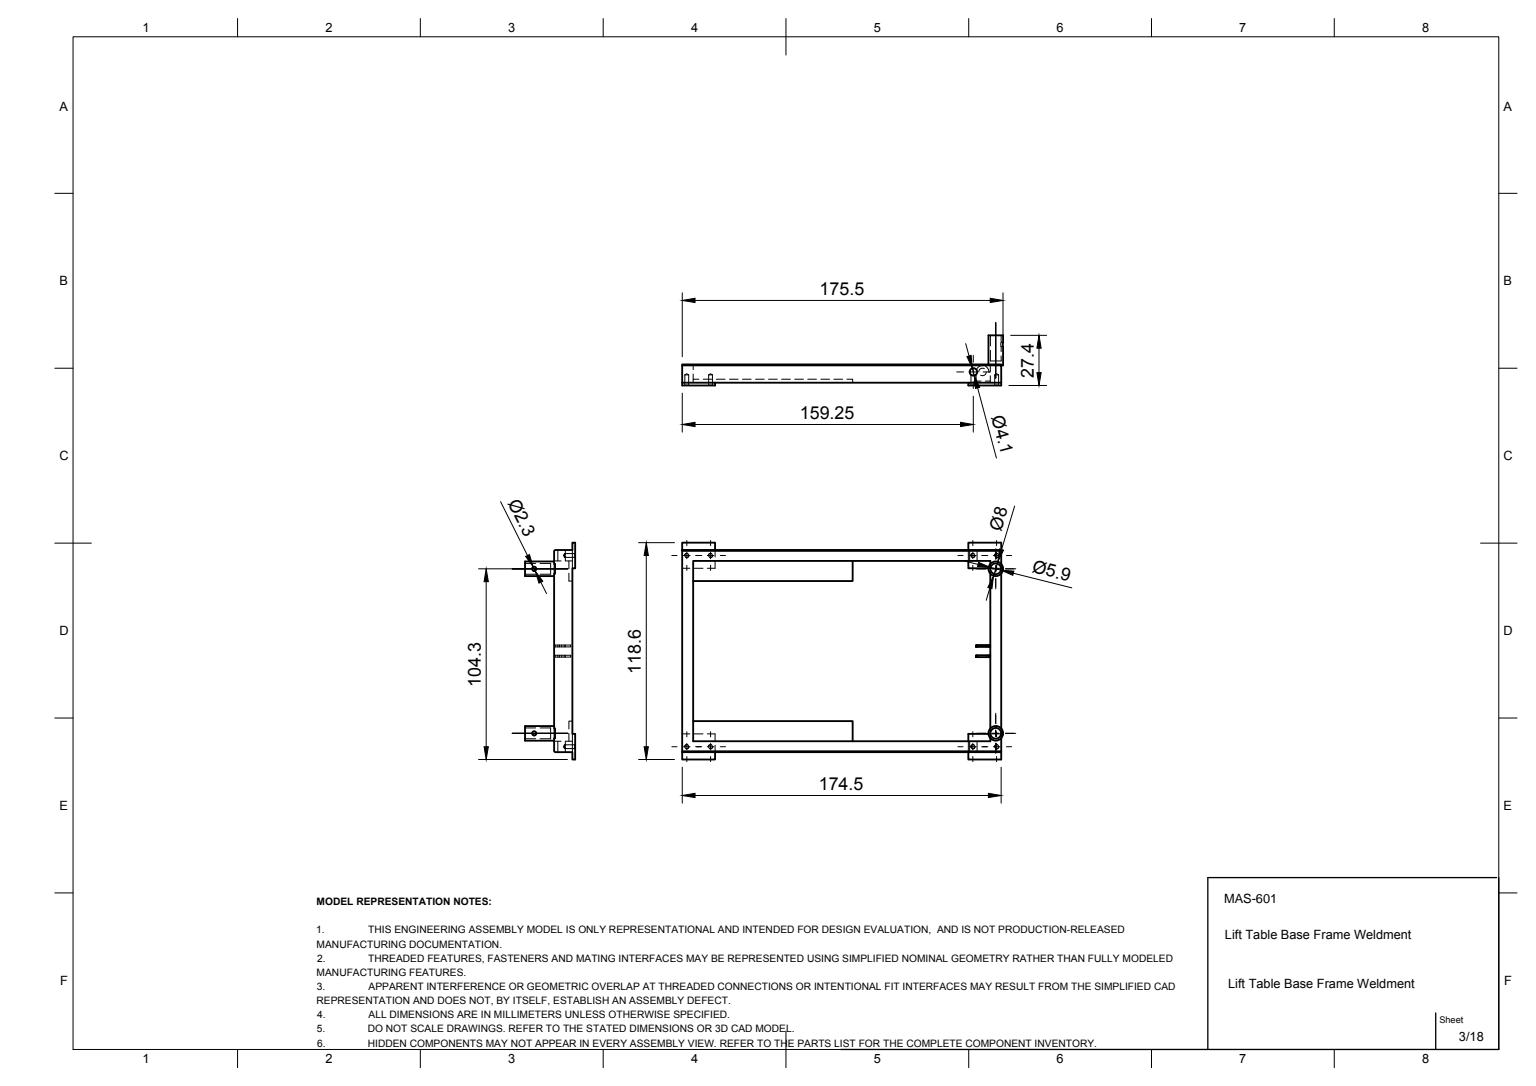
ISO-10303-21;
HEADER;
FILE_DESCRIPTION((''),'2;1');
FILE_NAME('Lift Table Base Frame Weldment.step','2026-10-06T07:37:42+05:00',(''),(''),'','','');
FILE_SCHEMA (('AUTOMOTIVE_DESIGN { 1 0 10303 214 3 1 1 }'));
ENDSEC;
DATA;
#10=MECHANICAL_DESIGN_GEOMETRIC_PRESENTATION_REPRESENTATION('',(#373),#18757);
#339=SHAPE_REPRESENTATION_RELATIONSHIP('SRR','None',#18857,#356) ;
#356=ADVANCED_BREP_SHAPE_REPRESENTATION('',(#390),#18740) ;
#373=STYLED_ITEM('',(#18951),#390) ;
#390=MANIFOLD_SOLID_BREP('Lift Table Base Frame Weldment',#9542) ;
#407=B_SPLINE_CURVE_WITH_KNOTS('',3,(#13518,#13519,#13520,#13521,#13522,
#13523,#13524,#13525,#13526,#13527,#13528,#13529,#13530,#13531,#13532,#13533,
#13534,#13535,#13536,#13537,#13538,#13539,#13540,#13541,#13542,#13543,#13544,
#13545,#13546,#13547,#13548,#13549,#13550,#13551,#13552),.UNSPECIFIED.,
 .F.,.F.,(4,2,2,2,2,2,2,2,3,2,2,2,2,2,2,2,4),(0.344577820460866,0.365980688401704,
0.406814525836436,0.448673337816236,0.490532149796036,0.530173091565364,
0.569814033334692,0.610053867634319,0.650293701933945,0.690533536233571,
0.730773370533197,0.770414312302526,0.810055254071854,0.851914066051654,
0.893772878031454,0.934606715466186,0.956009583407023),.UNSPECIFIED.) ;
#408=B_SPLINE_CURVE_WITH_KNOTS('',3,(#13564,#13565,#13566,#13567,#13568,
#13569,#13570,#13571,#13572,#13573,#13574,#13575,#13576,#13577,#13578,#13579,
#13580,#13581,#13582,#13583,#13584,#13585,#13586,#13587,#13588,#13589,#13590,
#13591,#13592,#13593,#13594,#13595,#13596,#13597,#13598),.UNSPECIFIED.,
 .F.,.F.,(4,2,2,2,2,2,2,2,3,2,2,2,2,2,2,2,4),(0.344577820460867,0.365980688401704,
0.406814525836436,0.448673337816236,0.490532149796036,0.530173091565364,
0.569814033334692,0.610053867634319,0.650293701933945,0.690533536233571,
0.730773370533197,0.770414312302526,0.810055254071854,0.851914066051654,
0.893772878031454,0.934606715466186,0.956009583407027),.UNSPECIFIED.) ;
#409=B_SPLINE_CURVE_WITH_KNOTS('',3,(#13629,#13630,#13631,#13632,#13633,
#13634,#13635),.UNSPECIFIED.,.F.,.F.,(4,3,4),(-0.0190556203788655,0.,0.0190556203788683),
 .UNSPECIFIED.) ;
#410=B_SPLINE_CURVE_WITH_KNOTS('',3,(#13646,#13647,#13648,#13649,#13650,
#13651,#13652),.UNSPECIFIED.,.F.,.F.,(4,3,4),(-0.019055620378868,0.,0.0190556203788661),
 .UNSPECIFIED.) ;
#411=B_SPLINE_CURVE_WITH_KNOTS('',3,(#13665,#13666,#13667,#13668,#13669,
#13670,#13671,#13672,#13673,#13674),.UNSPECIFIED.,.F.,.F.,(4,2,2,2,4),(0.,
0.0435910279952308,0.0871820559904617,0.130762210503654,0.174342365016846),
 .UNSPECIFIED.) ;
#412=B_SPLINE_CURVE_WITH_KNOTS('',3,(#13675,#13676,#13677,#13678,#13679,
#13680,#13681,#13682,#13683,#13684,#13685,#13686,#13687,#13688,#13689,#13690,
#13691,#13692,#13693,#13694,#13695,#13696,#13697,#13698,#13699,#13700),
 .UNSPECIFIED.,.F.,.F.,(4,2,2,2,2,2,2,2,2,2,2,2,4),(0.174342365016846,0.217922519530038,
0.261502674043231,0.305093702038462,0.348684730033692,0.392275758028923,
0.435866786024154,0.479446940537346,0.523027095050539,0.566607249563731,
0.610187404076923,0.653778432072154,0.697369460067385),.UNSPECIFIED.) ;
#413=B_SPLINE_CURVE_WITH_KNOTS('',3,(#13704,#13705,#13706,#13707,#13708,
#13709,#13710,#13711,#13712,#13713),.UNSPECIFIED.,.F.,.F.,(4,2,2,2,4),(0.,
0.0438474980267263,0.0876949960534527,0.131502815085544,0.175310634117636),
 .UNSPECIFIED.) ;
#414=B_SPLINE_CURVE_WITH_KNOTS('',3,(#13714,#13715,#13716,#13717,#13718,
#13719,#13720,#13721,#13722,#13723,#13724,#13725,#13726,#13727,#13728,#13729,
#13730,#13731,#13732,#13733,#13734,#13735,#13736,#13737,#13738,#13739),
 .UNSPECIFIED.,.F.,.F.,(4,2,2,2,2,2,2,2,2,2,2,2,4),(0.175310634117636,0.219118453149728,
0.26292627218182,0.306773770208546,0.350621268235272,0.394468766261999,
0.438316264288725,0.482124083320817,0.525931902352908,0.569739721385,0.613547540417092,
0.657395038443818,0.701242536470545),.UNSPECIFIED.) ;
#415=B_SPLINE_CURVE_WITH_KNOTS('',3,(#13750,#13751,#13752,#13753,#13754,
#13755,#13756,#13757,#13758,#13759),.UNSPECIFIED.,.F.,.F.,(4,2,2,2,4),(0.,
0.0435910279952308,0.0871820559904617,0.130762210503654,0.174342365016846),
 .UNSPECIFIED.) ;
#416=B_SPLINE_CURVE_WITH_KNOTS('',3,(#13760,#13761,#13762,#13763,#13764,
#13765,#13766,#13767,#13768,#13769,#13770,#13771,#13772,#13773,#13774,#13775,
#13776,#13777,#13778,#13779,#13780,#13781,#13782,#13783,#13784,#13785),
 .UNSPECIFIED.,.F.,.F.,(4,2,2,2,2,2,2,2,2,2,2,2,4),(0.174342365016846,0.217922519530038,
0.261502674043231,0.305093702038462,0.348684730033692,0.392275758028923,
0.435866786024154,0.479446940537346,0.523027095050539,0.566607249563731,
0.610187404076923,0.653778432072154,0.697369460067385),.UNSPECIFIED.) ;
#417=B_SPLINE_CURVE_WITH_KNOTS('',3,(#13789,#13790,#13791,#13792,#13793,
#13794,#13795,#13796,#13797,#13798),.UNSPECIFIED.,.F.,.F.,(4,2,2,2,4),(0.,
0.0438474980267263,0.0876949960534527,0.131502815085544,0.175310634117636),
 .UNSPECIFIED.) ;
#418=B_SPLINE_CURVE_WITH_KNOTS('',3,(#13799,#13800,#13801,#13802,#13803,
#13804,#13805,#13806,#13807,#13808,#13809,#13810,#13811,#13812,#13813,#13814,
#13815,#13816,#13817,#13818,#13819,#13820,#13821,#13822,#13823,#13824),
 .UNSPECIFIED.,.F.,.F.,(4,2,2,2,2,2,2,2,2,2,2,2,4),(0.175310634117636,0.219118453149728,
0.26292627218182,0.306773770208546,0.350621268235272,0.394468766261999,
0.438316264288725,0.482124083320817,0.525931902352908,0.569739721385,0.613547540417092,
0.657395038443818,0.701242536470545),.UNSPECIFIED.) ;
#500=CYLINDRICAL_SURFACE('',#9754,1.05) ;
#501=CYLINDRICAL_SURFACE('',#9761,1.05) ;
#502=CYLINDRICAL_SURFACE('',#9768,1.05) ;
#503=CYLINDRICAL_SURFACE('',#9775,1.05) ;
#504=CYLINDRICAL_SURFACE('',#9779,1.05) ;
#505=CYLINDRICAL_SURFACE('',#9784,1.05) ;
#506=CYLINDRICAL_SURFACE('',#9789,1.05) ;
#507=CYLINDRICAL_SURFACE('',#9793,1.05) ;
#508=CYLINDRICAL_SURFACE('',#9800,2.05) ;
#509=CYLINDRICAL_SURFACE('',#9805,2.05) ;
#510=CYLINDRICAL_SURFACE('',#9809,1.15) ;
#511=CYLINDRICAL_SURFACE('',#9810,2.95) ;
#512=CYLINDRICAL_SURFACE('',#9814,1.15) ;
#513=CYLINDRICAL_SURFACE('',#9815,2.95) ;
#514=CYLINDRICAL_SURFACE('',#9819,2.05) ;
#515=CYLINDRICAL_SURFACE('',#9822,2.05) ;
#516=CYLINDRICAL_SURFACE('',#9825,2.05) ;
#517=CYLINDRICAL_SURFACE('',#9828,2.05) ;
#518=CYLINDRICAL_SURFACE('',#9842,3.99999999999999) ;
#519=CYLINDRICAL_SURFACE('',#9857,3.50000000000001) ;
#520=CYLINDRICAL_SURFACE('',#9863,3.99999999999999) ;
#521=CYLINDRICAL_SURFACE('',#9874,3.50000000000001) ;
#651=FACE_BOUND('',#1608,.T.) ;
#652=FACE_BOUND('',#1609,.T.) ;
#653=FACE_BOUND('',#1613,.T.) ;
#654=FACE_BOUND('',#1614,.T.) ;
#655=FACE_BOUND('',#1618,.T.) ;
#656=FACE_BOUND('',#1619,.T.) ;
#657=FACE_BOUND('',#1623,.T.) ;
#658=FACE_BOUND('',#1624,.T.) ;
#659=FACE_BOUND('',#1640,.T.) ;
#660=FACE_BOUND('',#1644,.T.) ;
#661=FACE_BOUND('',#1648,.T.) ;
#662=FACE_BOUND('',#1652,.T.) ;
#663=FACE_BOUND('',#1660,.T.) ;
#664=FACE_BOUND('',#1663,.T.) ;
#665=FACE_BOUND('',#1666,.T.) ;
#666=FACE_BOUND('',#1670,.T.) ;
#667=FACE_BOUND('',#1672,.T.) ;
#668=FACE_BOUND('',#1676,.T.) ;
#669=FACE_BOUND('',#1678,.T.) ;
#670=FACE_BOUND('',#1679,.T.) ;
#671=FACE_BOUND('',#1685,.T.) ;
#672=FACE_BOUND('',#1690,.T.) ;
#673=FACE_BOUND('',#1694,.T.) ;
#674=FACE_BOUND('',#1699,.T.) ;
#675=FACE_BOUND('',#1714,.T.) ;
#676=FACE_BOUND('',#1727,.T.) ;
#759=PLANE('',#9752) ;
#760=PLANE('',#9759) ;
#761=PLANE('',#9766) ;
#762=PLANE('',#9773) ;
#763=PLANE('',#9813) ;
#764=PLANE('',#9818) ;
#765=PLANE('',#9831) ;
#766=PLANE('',#9832) ;
#767=PLANE('',#9834) ;
#768=PLANE('',#9835) ;
#769=PLANE('',#9837) ;
#770=PLANE('',#9838) ;
#771=PLANE('',#9839) ;
#772=PLANE('',#9840) ;
#773=PLANE('',#9841) ;
#774=PLANE('',#9849) ;
#775=PLANE('',#9850) ;
#776=PLANE('',#9851) ;
#777=PLANE('',#9852) ;
#778=PLANE('',#9853) ;
#779=PLANE('',#9855) ;
#780=PLANE('',#9856) ;
#781=PLANE('',#9859) ;
#782=PLANE('',#9860) ;
#783=PLANE('',#9861) ;
#784=PLANE('',#9862) ;
#785=PLANE('',#9869) ;
#786=PLANE('',#9870) ;
#787=PLANE('',#9871) ;
#788=PLANE('',#9872) ;
#789=PLANE('',#9873) ;
#790=PLANE('',#9876) ;
#791=PLANE('',#9877) ;
#792=PLANE('',#9878) ;
#793=PLANE('',#9879) ;
#794=PLANE('',#9880) ;
#795=PLANE('',#9881) ;
#796=PLANE('',#9882) ;
#797=PLANE('',#9883) ;
#798=PLANE('',#9884) ;
#799=PLANE('',#9885) ;
#800=PLANE('',#9886) ;
#801=PLANE('',#9887) ;
#802=PLANE('',#9888) ;
#803=PLANE('',#9889) ;
#804=PLANE('',#9890) ;
#805=PLANE('',#9891) ;
#806=PLANE('',#9892) ;
#807=PLANE('',#9893) ;
#808=PLANE('',#9894) ;
#809=PLANE('',#9895) ;
#810=PLANE('',#9896) ;
#811=PLANE('',#9897) ;
#812=PLANE('',#9898) ;
#813=PLANE('',#9899) ;
#814=PLANE('',#9900) ;
#815=PLANE('',#9901) ;
#816=PLANE('',#9902) ;
#817=PLANE('',#9903) ;
#818=PLANE('',#9904) ;
#1087=FACE_OUTER_BOUND('',#1606,.T.) ;
#1088=FACE_OUTER_BOUND('',#1607,.T.) ;
#1089=FACE_OUTER_BOUND('',#1610,.T.) ;
#1090=FACE_OUTER_BOUND('',#1611,.T.) ;
#1091=FACE_OUTER_BOUND('',#1612,.T.) ;
#1092=FACE_OUTER_BOUND('',#1615,.T.) ;
#1093=FACE_OUTER_BOUND('',#1616,.T.) ;
#1094=FACE_OUTER_BOUND('',#1617,.T.) ;
#1095=FACE_OUTER_BOUND('',#1620,.T.) ;
#1096=FACE_OUTER_BOUND('',#1621,.T.) ;
#1097=FACE_OUTER_BOUND('',#1622,.T.) ;
#1098=FACE_OUTER_BOUND('',#1625,.T.) ;
#1099=FACE_OUTER_BOUND('',#1626,.T.) ;
#1100=FACE_OUTER_BOUND('',#1627,.T.) ;
#1101=FACE_OUTER_BOUND('',#1628,.T.) ;
#1102=FACE_OUTER_BOUND('',#1629,.T.) ;
#1103=FACE_OUTER_BOUND('',#1630,.T.) ;
#1104=FACE_OUTER_BOUND('',#1631,.T.) ;
#1105=FACE_OUTER_BOUND('',#1632,.T.) ;
#1106=FACE_OUTER_BOUND('',#1633,.T.) ;
#1107=FACE_OUTER_BOUND('',#1634,.T.) ;
#1108=FACE_OUTER_BOUND('',#1635,.T.) ;
#1109=FACE_OUTER_BOUND('',#1636,.T.) ;
#1110=FACE_OUTER_BOUND('',#1637,.T.) ;
#1111=FACE_OUTER_BOUND('',#1638,.T.) ;
#1112=FACE_OUTER_BOUND('',#1639,.T.) ;
#1113=FACE_OUTER_BOUND('',#1641,.T.) ;
#1114=FACE_OUTER_BOUND('',#1642,.T.) ;
#1115=FACE_OUTER_BOUND('',#1643,.T.) ;
#1116=FACE_OUTER_BOUND('',#1645,.T.) ;
#1117=FACE_OUTER_BOUND('',#1646,.T.) ;
#1118=FACE_OUTER_BOUND('',#1647,.T.) ;
#1119=FACE_OUTER_BOUND('',#1649,.T.) ;
#1120=FACE_OUTER_BOUND('',#1650,.T.) ;
#1121=FACE_OUTER_BOUND('',#1651,.T.) ;
#1122=FACE_OUTER_BOUND('',#1653,.T.) ;
#1123=FACE_OUTER_BOUND('',#1654,.T.) ;
#1124=FACE_OUTER_BOUND('',#1655,.T.) ;
#1125=FACE_OUTER_BOUND('',#1656,.T.) ;
#1126=FACE_OUTER_BOUND('',#1657,.T.) ;
#1127=FACE_OUTER_BOUND('',#1658,.T.) ;
#1128=FACE_OUTER_BOUND('',#1659,.T.) ;
#1129=FACE_OUTER_BOUND('',#1661,.T.) ;
#1130=FACE_OUTER_BOUND('',#1662,.T.) ;
#1131=FACE_OUTER_BOUND('',#1664,.T.) ;
#1132=FACE_OUTER_BOUND('',#1665,.T.) ;
#1133=FACE_OUTER_BOUND('',#1667,.T.) ;
#1134=FACE_OUTER_BOUND('',#1668,.T.) ;
#1135=FACE_OUTER_BOUND('',#1669,.T.) ;
#1136=FACE_OUTER_BOUND('',#1671,.T.) ;
#1137=FACE_OUTER_BOUND('',#1673,.T.) ;
#1138=FACE_OUTER_BOUND('',#1674,.T.) ;
#1139=FACE_OUTER_BOUND('',#1675,.T.) ;
#1140=FACE_OUTER_BOUND('',#1677,.T.) ;
#1141=FACE_OUTER_BOUND('',#1680,.T.) ;
#1142=FACE_OUTER_BOUND('',#1681,.T.) ;
#1143=FACE_OUTER_BOUND('',#1682,.T.) ;
#1144=FACE_OUTER_BOUND('',#1683,.T.) ;
#1145=FACE_OUTER_BOUND('',#1684,.T.) ;
#1146=FACE_OUTER_BOUND('',#1686,.T.) ;
#1147=FACE_OUTER_BOUND('',#1687,.T.) ;
#1148=FACE_OUTER_BOUND('',#1688,.T.) ;
#1149=FACE_OUTER_BOUND('',#1689,.T.) ;
#1150=FACE_OUTER_BOUND('',#1691,.T.) ;
#1151=FACE_OUTER_BOUND('',#1692,.T.) ;
#1152=FACE_OUTER_BOUND('',#1693,.T.) ;
#1153=FACE_OUTER_BOUND('',#1695,.T.) ;
#1154=FACE_OUTER_BOUND('',#1696,.T.) ;
#1155=FACE_OUTER_BOUND('',#1697,.T.) ;
#1156=FACE_OUTER_BOUND('',#1698,.T.) ;
#1157=FACE_OUTER_BOUND('',#1700,.T.) ;
#1158=FACE_OUTER_BOUND('',#1701,.T.) ;
#1159=FACE_OUTER_BOUND('',#1702,.T.) ;
#1160=FACE_OUTER_BOUND('',#1703,.T.) ;
#1161=FACE_OUTER_BOUND('',#1704,.T.) ;
#1162=FACE_OUTER_BOUND('',#1705,.T.) ;
#1163=FACE_OUTER_BOUND('',#1706,.T.) ;
#1164=FACE_OUTER_BOUND('',#1707,.T.) ;
#1165=FACE_OUTER_BOUND('',#1708,.T.) ;
#1166=FACE_OUTER_BOUND('',#1709,.T.) ;
#1167=FACE_OUTER_BOUND('',#1710,.T.) ;
#1168=FACE_OUTER_BOUND('',#1711,.T.) ;
#1169=FACE_OUTER_BOUND('',#1712,.T.) ;
#1170=FACE_OUTER_BOUND('',#1713,.T.) ;
#1171=FACE_OUTER_BOUND('',#1715,.T.) ;
#1172=FACE_OUTER_BOUND('',#1716,.T.) ;
#1173=FACE_OUTER_BOUND('',#1717,.T.) ;
#1174=FACE_OUTER_BOUND('',#1718,.T.) ;
#1175=FACE_OUTER_BOUND('',#1719,.T.) ;
#1176=FACE_OUTER_BOUND('',#1720,.T.) ;
#1177=FACE_OUTER_BOUND('',#1721,.T.) ;
#1178=FACE_OUTER_BOUND('',#1722,.T.) ;
#1179=FACE_OUTER_BOUND('',#1723,.T.) ;
#1180=FACE_OUTER_BOUND('',#1724,.T.) ;
#1181=FACE_OUTER_BOUND('',#1725,.T.) ;
#1182=FACE_OUTER_BOUND('',#1726,.T.) ;
#1183=FACE_OUTER_BOUND('',#1728,.T.) ;
#1184=FACE_OUTER_BOUND('',#1729,.T.) ;
#1606=EDGE_LOOP('',(#6343,#6344,#6345,#6346)) ;
#1607=EDGE_LOOP('',(#6347,#6348,#6349,#6350)) ;
#1608=EDGE_LOOP('',(#6351)) ;
#1609=EDGE_LOOP('',(#6352)) ;
#1610=EDGE_LOOP('',(#6353,#6354,#6355,#6356)) ;
#1611=EDGE_LOOP('',(#6357,#6358,#6359,#6360)) ;
#1612=EDGE_LOOP('',(#6361,#6362,#6363,#6364)) ;
#1613=EDGE_LOOP('',(#6365)) ;
#1614=EDGE_LOOP('',(#6366)) ;
#1615=EDGE_LOOP('',(#6367,#6368,#6369,#6370)) ;
#1616=EDGE_LOOP('',(#6371,#6372,#6373,#6374)) ;
#1617=EDGE_LOOP('',(#6375,#6376,#6377,#6378)) ;
#1618=EDGE_LOOP('',(#6379)) ;
#1619=EDGE_LOOP('',(#6380)) ;
#1620=EDGE_LOOP('',(#6381,#6382,#6383,#6384)) ;
#1621=EDGE_LOOP('',(#6385,#6386,#6387,#6388)) ;
#1622=EDGE_LOOP('',(#6389,#6390,#6391,#6392)) ;
#1623=EDGE_LOOP('',(#6393)) ;
#1624=EDGE_LOOP('',(#6394)) ;
#1625=EDGE_LOOP('',(#6395,#6396,#6397,#6398)) ;
#1626=EDGE_LOOP('',(#6399,#6400,#6401,#6402)) ;
#1627=EDGE_LOOP('',(#6403,#6404,#6405,#6406,#6407,#6408)) ;
#1628=EDGE_LOOP('',(#6409,#6410,#6411,#6412)) ;
#1629=EDGE_LOOP('',(#6413,#6414,#6415,#6416,#6417,#6418)) ;
#1630=EDGE_LOOP('',(#6419,#6420,#6421,#6422)) ;
#1631=EDGE_LOOP('',(#6423,#6424,#6425,#6426)) ;
#1632=EDGE_LOOP('',(#6427,#6428,#6429,#6430)) ;
#1633=EDGE_LOOP('',(#6431,#6432,#6433,#6434)) ;
#1634=EDGE_LOOP('',(#6435,#6436,#6437)) ;
#1635=EDGE_LOOP('',(#6438,#6439,#6440)) ;
#1636=EDGE_LOOP('',(#6441,#6442,#6443)) ;
#1637=EDGE_LOOP('',(#6444,#6445,#6446)) ;
#1638=EDGE_LOOP('',(#6447,#6448,#6449)) ;
#1639=EDGE_LOOP('',(#6450,#6451,#6452,#6453)) ;
#1640=EDGE_LOOP('',(#6454,#6455)) ;
#1641=EDGE_LOOP('',(#6456,#6457,#6458)) ;
#1642=EDGE_LOOP('',(#6459,#6460,#6461)) ;
#1643=EDGE_LOOP('',(#6462,#6463,#6464,#6465)) ;
#1644=EDGE_LOOP('',(#6466,#6467)) ;
#1645=EDGE_LOOP('',(#6468,#6469,#6470)) ;
#1646=EDGE_LOOP('',(#6471,#6472,#6473,#6474,#6475,#6476)) ;
#1647=EDGE_LOOP('',(#6477,#6478,#6479,#6480)) ;
#1648=EDGE_LOOP('',(#6481,#6482)) ;
#1649=EDGE_LOOP('',(#6483)) ;
#1650=EDGE_LOOP('',(#6484,#6485,#6486,#6487,#6488,#6489)) ;
#1651=EDGE_LOOP('',(#6490,#6491,#6492,#6493)) ;
#1652=EDGE_LOOP('',(#6494,#6495)) ;
#1653=EDGE_LOOP('',(#6496)) ;
#1654=EDGE_LOOP('',(#6497,#6498,#6499,#6500)) ;
#1655=EDGE_LOOP('',(#6501,#6502,#6503,#6504)) ;
#1656=EDGE_LOOP('',(#6505,#6506,#6507,#6508)) ;
#1657=EDGE_LOOP('',(#6509,#6510,#6511,#6512)) ;
#1658=EDGE_LOOP('',(#6513,#6514,#6515,#6516)) ;
#1659=EDGE_LOOP('',(#6517,#6518,#6519,#6520,#6521,#6522)) ;
#1660=EDGE_LOOP('',(#6523)) ;
#1661=EDGE_LOOP('',(#6524,#6525,#6526,#6527)) ;
#1662=EDGE_LOOP('',(#6528,#6529,#6530,#6531,#6532,#6533)) ;
#1663=EDGE_LOOP('',(#6534)) ;
#1664=EDGE_LOOP('',(#6535,#6536,#6537,#6538)) ;
#1665=EDGE_LOOP('',(#6539,#6540,#6541,#6542,#6543,#6544)) ;
#1666=EDGE_LOOP('',(#6545)) ;
#1667=EDGE_LOOP('',(#6546,#6547,#6548,#6549,#6550,#6551,#6552,#6553,#6554,
#6555,#6556,#6557,#6558,#6559,#6560,#6561,#6562,#6563,#6564,#6565,#6566,
#6567)) ;
#1668=EDGE_LOOP('',(#6568,#6569,#6570,#6571)) ;
#1669=EDGE_LOOP('',(#6572,#6573,#6574,#6575,#6576,#6577)) ;
#1670=EDGE_LOOP('',(#6578)) ;
#1671=EDGE_LOOP('',(#6579,#6580,#6581,#6582,#6583,#6584,#6585,#6586,#6587,
#6588,#6589,#6590)) ;
#1672=EDGE_LOOP('',(#6591,#6592)) ;
#1673=EDGE_LOOP('',(#6593,#6594)) ;
#1674=EDGE_LOOP('',(#6595,#6596,#6597)) ;
#1675=EDGE_LOOP('',(#6598)) ;
#1676=EDGE_LOOP('',(#6599)) ;
#1677=EDGE_LOOP('',(#6600,#6601,#6602,#6603,#6604,#6605,#6606,#6607,#6608,
#6609,#6610,#6611,#6612,#6613)) ;
#1678=EDGE_LOOP('',(#6614,#6615,#6616,#6617)) ;
#1679=EDGE_LOOP('',(#6618,#6619,#6620,#6621)) ;
#1680=EDGE_LOOP('',(#6622,#6623,#6624,#6625)) ;
#1681=EDGE_LOOP('',(#6626,#6627,#6628,#6629)) ;
#1682=EDGE_LOOP('',(#6630,#6631,#6632,#6633)) ;
#1683=EDGE_LOOP('',(#6634,#6635,#6636,#6637)) ;
#1684=EDGE_LOOP('',(#6638,#6639,#6640,#6641,#6642,#6643)) ;
#1685=EDGE_LOOP('',(#6644)) ;
#1686=EDGE_LOOP('',(#6645,#6646,#6647,#6648)) ;
#1687=EDGE_LOOP('',(#6649,#6650,#6651,#6652)) ;
#1688=EDGE_LOOP('',(#6653,#6654,#6655,#6656)) ;
#1689=EDGE_LOOP('',(#6657,#6658,#6659,#6660,#6661,#6662,#6663,#6664,#6665,
#6666,#6667,#6668)) ;
#1690=EDGE_LOOP('',(#6669,#6670)) ;
#1691=EDGE_LOOP('',(#6671,#6672)) ;
#1692=EDGE_LOOP('',(#6673,#6674,#6675)) ;
#1693=EDGE_LOOP('',(#6676)) ;
#1694=EDGE_LOOP('',(#6677)) ;
#1695=EDGE_LOOP('',(#6678,#6679,#6680,#6681)) ;
#1696=EDGE_LOOP('',(#6682,#6683,#6684,#6685)) ;
#1697=EDGE_LOOP('',(#6686,#6687,#6688,#6689)) ;
#1698=EDGE_LOOP('',(#6690,#6691,#6692,#6693,#6694,#6695)) ;
#1699=EDGE_LOOP('',(#6696)) ;
#1700=EDGE_LOOP('',(#6697,#6698,#6699,#6700)) ;
#1701=EDGE_LOOP('',(#6701,#6702,#6703,#6704)) ;
#1702=EDGE_LOOP('',(#6705,#6706,#6707,#6708)) ;
#1703=EDGE_LOOP('',(#6709,#6710,#6711,#6712)) ;
#1704=EDGE_LOOP('',(#6713,#6714,#6715,#6716)) ;
#1705=EDGE_LOOP('',(#6717,#6718,#6719,#6720,#6721)) ;
#1706=EDGE_LOOP('',(#6722,#6723,#6724,#6725)) ;
#1707=EDGE_LOOP('',(#6726,#6727,#6728,#6729)) ;
#1708=EDGE_LOOP('',(#6730,#6731,#6732,#6733)) ;
#1709=EDGE_LOOP('',(#6734,#6735,#6736,#6737,#6738)) ;
#1710=EDGE_LOOP('',(#6739,#6740,#6741,#6742)) ;
#1711=EDGE_LOOP('',(#6743,#6744,#6745,#6746,#6747,#6748,#6749,#6750,#6751,
#6752,#6753,#6754,#6755,#6756,#6757,#6758)) ;
#1712=EDGE_LOOP('',(#6759,#6760,#6761,#6762,#6763,#6764,#6765,#6766)) ;
#1713=EDGE_LOOP('',(#6767,#6768,#6769,#6770,#6771,#6772,#6773)) ;
#1714=EDGE_LOOP('',(#6774)) ;
#1715=EDGE_LOOP('',(#6775,#6776,#6777,#6778)) ;
#1716=EDGE_LOOP('',(#6779,#6780,#6781,#6782,#6783)) ;
#1717=EDGE_LOOP('',(#6784,#6785,#6786,#6787)) ;
#1718=EDGE_LOOP('',(#6788,#6789,#6790,#6791,#6792,#6793)) ;
#1719=EDGE_LOOP('',(#6794,#6795,#6796,#6797)) ;
#1720=EDGE_LOOP('',(#6798,#6799,#6800,#6801)) ;
#1721=EDGE_LOOP('',(#6802,#6803,#6804,#6805)) ;
#1722=EDGE_LOOP('',(#6806,#6807,#6808,#6809)) ;
#1723=EDGE_LOOP('',(#6810,#6811,#6812,#6813)) ;
#1724=EDGE_LOOP('',(#6814,#6815,#6816,#6817,#6818)) ;
#1725=EDGE_LOOP('',(#6819,#6820,#6821,#6822,#6823,#6824)) ;
#1726=EDGE_LOOP('',(#6825,#6826,#6827,#6828,#6829,#6830,#6831)) ;
#1727=EDGE_LOOP('',(#6832)) ;
#1728=EDGE_LOOP('',(#6833,#6834,#6835,#6836,#6837,#6838,#6839,#6840,#6841,
#6842,#6843,#6844,#6845,#6846)) ;
#1729=EDGE_LOOP('',(#6847,#6848,#6849,#6850,#6851,#6852,#6853,#6854,#6855,
#6856,#6857,#6858)) ;
#2233=LINE('',#13428,#3004) ;
#2234=LINE('',#13433,#3005) ;
#2235=LINE('',#13435,#3006) ;
#2236=LINE('',#13437,#3007) ;
#2237=LINE('',#13438,#3008) ;
#2238=LINE('',#13443,#3009) ;
#2239=LINE('',#13449,#3010) ;
#2240=LINE('',#13454,#3011) ;
#2241=LINE('',#13456,#3012) ;
#2242=LINE('',#13458,#3013) ;
#2243=LINE('',#13459,#3014) ;
#2244=LINE('',#13464,#3015) ;
#2245=LINE('',#13470,#3016) ;
#2246=LINE('',#13475,#3017) ;
#2247=LINE('',#13477,#3018) ;
#2248=LINE('',#13479,#3019) ;
#2249=LINE('',#13480,#3020) ;
#2250=LINE('',#13485,#3021) ;
#2251=LINE('',#13491,#3022) ;
#2252=LINE('',#13496,#3023) ;
#2253=LINE('',#13498,#3024) ;
#2254=LINE('',#13500,#3025) ;
#2255=LINE('',#13501,#3026) ;
#2256=LINE('',#13506,#3027) ;
#2257=LINE('',#13510,#3028) ;
#2258=LINE('',#13514,#3029) ;
#2259=LINE('',#13556,#3030) ;
#2260=LINE('',#13560,#3031) ;
#2261=LINE('',#13602,#3032) ;
#2262=LINE('',#13606,#3033) ;
#2263=LINE('',#13610,#3034) ;
#2264=LINE('',#13614,#3035) ;
#2265=LINE('',#13618,#3036) ;
#2266=LINE('',#13621,#3037) ;
#2267=LINE('',#13624,#3038) ;
#2268=LINE('',#13627,#3039) ;
#2269=LINE('',#13640,#3040) ;
#2270=LINE('',#13644,#3041) ;
#2271=LINE('',#13657,#3042) ;
#2272=LINE('',#13661,#3043) ;
#2273=LINE('',#13702,#3044) ;
#2274=LINE('',#13744,#3045) ;
#2275=LINE('',#13787,#3046) ;
#2276=LINE('',#13829,#3047) ;
#2277=LINE('',#13836,#3048) ;
#2278=LINE('',#13842,#3049) ;
#2279=LINE('',#13847,#3050) ;
#2280=LINE('',#13851,#3051) ;
#2281=LINE('',#13856,#3052) ;
#2282=LINE('',#13860,#3053) ;
#2283=LINE('',#13864,#3054) ;
#2284=LINE('',#13866,#3055) ;
#2285=LINE('',#13867,#3056) ;
#2286=LINE('',#13872,#3057) ;
#2287=LINE('',#13874,#3058) ;
#2288=LINE('',#13875,#3059) ;
#2289=LINE('',#13878,#3060) ;
#2290=LINE('',#13880,#3061) ;
#2291=LINE('',#13881,#3062) ;
#2292=LINE('',#13886,#3063) ;
#2293=LINE('',#13888,#3064) ;
#2294=LINE('',#13889,#3065) ;
#2295=LINE('',#13893,#3066) ;
#2296=LINE('',#13895,#3067) ;
#2297=LINE('',#13897,#3068) ;
#2298=LINE('',#13898,#3069) ;
#2299=LINE('',#13901,#3070) ;
#2300=LINE('',#13903,#3071) ;
#2301=LINE('',#13905,#3072) ;
#2302=LINE('',#13907,#3073) ;
#2303=LINE('',#13908,#3074) ;
#2304=LINE('',#13911,#3075) ;
#2305=LINE('',#13913,#3076) ;
#2306=LINE('',#13915,#3077) ;
#2307=LINE('',#13917,#3078) ;
#2308=LINE('',#13919,#3079) ;
#2309=LINE('',#13921,#3080) ;
#2310=LINE('',#13923,#3081) ;
#2311=LINE('',#13925,#3082) ;
#2312=LINE('',#13927,#3083) ;
#2313=LINE('',#13929,#3084) ;
#2314=LINE('',#13931,#3085) ;
#2315=LINE('',#13933,#3086) ;
#2316=LINE('',#13934,#3087) ;
#2317=LINE('',#13936,#3088) ;
#2318=LINE('',#13938,#3089) ;
#2319=LINE('',#13939,#3090) ;
#2320=LINE('',#13941,#3091) ;
#2321=LINE('',#13942,#3092) ;
#2322=LINE('',#13945,#3093) ;
#2323=LINE('',#13947,#3094) ;
#2324=LINE('',#13948,#3095) ;
#2325=LINE('',#13951,#3096) ;
#2326=LINE('',#13953,#3097) ;
#2327=LINE('',#13955,#3098) ;
#2328=LINE('',#13956,#3099) ;
#2329=LINE('',#13961,#3100) ;
#2330=LINE('',#13965,#3101) ;
#2331=LINE('',#13971,#3102) ;
#2332=LINE('',#13975,#3103) ;
#2333=LINE('',#13979,#3104) ;
#2334=LINE('',#13981,#3105) ;
#2335=LINE('',#13983,#3106) ;
#2336=LINE('',#13985,#3107) ;
#2337=LINE('',#13987,#3108) ;
#2338=LINE('',#13989,#3109) ;
#2339=LINE('',#13991,#3110) ;
#2340=LINE('',#13993,#3111) ;
#2341=LINE('',#13995,#3112) ;
#2342=LINE('',#13997,#3113) ;
#2343=LINE('',#13998,#3114) ;
#2344=LINE('',#14000,#3115) ;
#2345=LINE('',#14002,#3116) ;
#2346=LINE('',#14003,#3117) ;
#2347=LINE('',#14005,#3118) ;
#2348=LINE('',#14007,#3119) ;
#2349=LINE('',#14008,#3120) ;
#2350=LINE('',#14012,#3121) ;
#2351=LINE('',#14015,#3122) ;
#2352=LINE('',#14016,#3123) ;
#2353=LINE('',#14023,#3124) ;
#2354=LINE('',#14025,#3125) ;
#2355=LINE('',#14027,#3126) ;
#2356=LINE('',#14028,#3127) ;
#2357=LINE('',#14031,#3128) ;
#2358=LINE('',#14033,#3129) ;
#2359=LINE('',#14034,#3130) ;
#2360=LINE('',#14037,#3131) ;
#2361=LINE('',#14038,#3132) ;
#2362=LINE('',#14043,#3133) ;
#2363=LINE('',#14052,#3134) ;
#2364=LINE('',#14055,#3135) ;
#2365=LINE('',#14056,#3136) ;
#2366=LINE('',#14063,#3137) ;
#2367=LINE('',#14065,#3138) ;
#2368=LINE('',#14067,#3139) ;
#2369=LINE('',#14068,#3140) ;
#2370=LINE('',#14071,#3141) ;
#2371=LINE('',#14073,#3142) ;
#2372=LINE('',#14074,#3143) ;
#2373=LINE('',#14077,#3144) ;
#2374=LINE('',#14078,#3145) ;
#2375=LINE('',#14081,#3146) ;
#2376=LINE('',#14083,#3147) ;
#2377=LINE('',#14084,#3148) ;
#2378=LINE('',#14087,#3149) ;
#2379=LINE('',#14089,#3150) ;
#2380=LINE('',#14090,#3151) ;
#2381=LINE('',#14092,#3152) ;
#2382=LINE('',#14093,#3153) ;
#2383=LINE('',#14095,#3154) ;
#2384=LINE('',#14098,#3155) ;
#2385=LINE('',#14100,#3156) ;
#2386=LINE('',#14101,#3157) ;
#2387=LINE('',#14103,#3158) ;
#2388=LINE('',#14104,#3159) ;
#2389=LINE('',#14107,#3160) ;
#2390=LINE('',#14108,#3161) ;
#2391=LINE('',#14111,#3162) ;
#2392=LINE('',#14112,#3163) ;
#2393=LINE('',#14114,#3164) ;
#2394=LINE('',#14116,#3165) ;
#2395=LINE('',#14117,#3166) ;
#2396=LINE('',#14118,#3167) ;
#2397=LINE('',#14120,#3168) ;
#2398=LINE('',#14121,#3169) ;
#2399=LINE('',#14124,#3170) ;
#2400=LINE('',#14126,#3171) ;
#2401=LINE('',#14127,#3172) ;
#2402=LINE('',#14129,#3173) ;
#2403=LINE('',#14130,#3174) ;
#2404=LINE('',#14133,#3175) ;
#2405=LINE('',#14134,#3176) ;
#2406=LINE('',#14137,#3177) ;
#2407=LINE('',#14138,#3178) ;
#2408=LINE('',#14139,#3179) ;
#2409=LINE('',#14141,#3180) ;
#2410=LINE('',#14143,#3181) ;
#2411=LINE('',#14145,#3182) ;
#2412=LINE('',#14147,#3183) ;
#2413=LINE('',#14150,#3184) ;
#2414=LINE('',#14151,#3185) ;
#2415=LINE('',#14154,#3186) ;
#2416=LINE('',#14155,#3187) ;
#2417=LINE('',#14157,#3188) ;
#2418=LINE('',#14159,#3189) ;
#2419=LINE('',#14162,#3190) ;
#2420=LINE('',#14164,#3191) ;
#3004=VECTOR('',#10723,1.12500000000001) ;
#3005=VECTOR('',#10728,10.) ;
#3006=VECTOR('',#10729,10.) ;
#3007=VECTOR('',#10730,10.) ;
#3008=VECTOR('',#10731,10.) ;
#3009=VECTOR('',#10736,1.05) ;
#3010=VECTOR('',#10743,1.12500000000001) ;
#3011=VECTOR('',#10748,10.) ;
#3012=VECTOR('',#10749,10.) ;
#3013=VECTOR('',#10750,10.) ;
#3014=VECTOR('',#10751,10.) ;
#3015=VECTOR('',#10756,1.05) ;
#3016=VECTOR('',#10763,1.12500000000001) ;
#3017=VECTOR('',#10768,10.) ;
#3018=VECTOR('',#10769,10.) ;
#3019=VECTOR('',#10770,10.) ;
#3020=VECTOR('',#10771,10.) ;
#3021=VECTOR('',#10776,1.05) ;
#3022=VECTOR('',#10783,1.12500000000001) ;
#3023=VECTOR('',#10788,10.) ;
#3024=VECTOR('',#10789,10.) ;
#3025=VECTOR('',#10790,10.) ;
#3026=VECTOR('',#10791,10.) ;
#3027=VECTOR('',#10796,1.05) ;
#3028=VECTOR('',#10801,1.125) ;
#3029=VECTOR('',#10806,1.05) ;
#3030=VECTOR('',#10813,1.125) ;
#3031=VECTOR('',#10818,1.05) ;
#3032=VECTOR('',#10825,1.125) ;
#3033=VECTOR('',#10830,1.05) ;
#3034=VECTOR('',#10835,1.125) ;
#3035=VECTOR('',#10840,1.05) ;
#3036=VECTOR('',#10845,1.04999999999999) ;
#3037=VECTOR('',#10848,1.05) ;
#3038=VECTOR('',#10851,1.04999999999999) ;
#3039=VECTOR('',#10854,1.05) ;
#3040=VECTOR('',#10861,2.05) ;
#3041=VECTOR('',#10866,1.05) ;
#3042=VECTOR('',#10873,2.05) ;
#3043=VECTOR('',#10878,1.05) ;
#3044=VECTOR('',#10881,1.15) ;
#3045=VECTOR('',#10886,2.95) ;
#3046=VECTOR('',#10893,1.15) ;
#3047=VECTOR('',#10898,2.95) ;
#3048=VECTOR('',#10907,2.05) ;
#3049=VECTOR('',#10914,2.05) ;
#3050=VECTOR('',#10919,10.) ;
#3051=VECTOR('',#10922,10.) ;
#3052=VECTOR('',#10927,10.) ;
#3053=VECTOR('',#10930,10.) ;
#3054=VECTOR('',#10935,10.) ;
#3055=VECTOR('',#10936,10.) ;
#3056=VECTOR('',#10937,10.) ;
#3057=VECTOR('',#10942,10.) ;
#3058=VECTOR('',#10943,10.) ;
#3059=VECTOR('',#10944,10.) ;
#3060=VECTOR('',#10947,10.) ;
#3061=VECTOR('',#10948,10.) ;
#3062=VECTOR('',#10949,10.) ;
#3063=VECTOR('',#10954,10.) ;
#3064=VECTOR('',#10955,10.) ;
#3065=VECTOR('',#10956,10.) ;
#3066=VECTOR('',#10959,10.) ;
#3067=VECTOR('',#10960,10.) ;
#3068=VECTOR('',#10961,10.) ;
#3069=VECTOR('',#10962,10.) ;
#3070=VECTOR('',#10965,10.) ;
#3071=VECTOR('',#10966,10.) ;
#3072=VECTOR('',#10967,10.) ;
#3073=VECTOR('',#10968,10.) ;
#3074=VECTOR('',#10969,10.) ;
#3075=VECTOR('',#10972,10.) ;
#3076=VECTOR('',#10973,10.) ;
#3077=VECTOR('',#10974,10.) ;
#3078=VECTOR('',#10975,10.) ;
#3079=VECTOR('',#10976,10.) ;
#3080=VECTOR('',#10977,10.) ;
#3081=VECTOR('',#10978,10.) ;
#3082=VECTOR('',#10979,10.) ;
#3083=VECTOR('',#10980,10.) ;
#3084=VECTOR('',#10981,10.) ;
#3085=VECTOR('',#10982,10.) ;
#3086=VECTOR('',#10983,10.) ;
#3087=VECTOR('',#10984,10.) ;
#3088=VECTOR('',#10985,10.) ;
#3089=VECTOR('',#10986,10.) ;
#3090=VECTOR('',#10987,10.) ;
#3091=VECTOR('',#10988,10.) ;
#3092=VECTOR('',#10989,10.) ;
#3093=VECTOR('',#10992,10.) ;
#3094=VECTOR('',#10993,10.) ;
#3095=VECTOR('',#10994,10.) ;
#3096=VECTOR('',#10997,10.) ;
#3097=VECTOR('',#10998,10.) ;
#3098=VECTOR('',#10999,10.) ;
#3099=VECTOR('',#11000,10.) ;
#3100=VECTOR('',#11005,3.99999999999999) ;
#3101=VECTOR('',#11008,10.) ;
#3102=VECTOR('',#11015,10.) ;
#3103=VECTOR('',#11022,10.) ;
#3104=VECTOR('',#11027,10.) ;
#3105=VECTOR('',#11028,10.) ;
#3106=VECTOR('',#11029,10.) ;
#3107=VECTOR('',#11030,10.) ;
#3108=VECTOR('',#11031,10.) ;
#3109=VECTOR('',#11032,10.) ;
#3110=VECTOR('',#11033,10.) ;
#3111=VECTOR('',#11034,10.) ;
#3112=VECTOR('',#11035,10.) ;
#3113=VECTOR('',#11036,10.) ;
#3114=VECTOR('',#11037,10.) ;
#3115=VECTOR('',#11038,10.) ;
#3116=VECTOR('',#11039,10.) ;
#3117=VECTOR('',#11040,10.) ;
#3118=VECTOR('',#11041,10.) ;
#3119=VECTOR('',#11042,10.) ;
#3120=VECTOR('',#11043,10.) ;
#3121=VECTOR('',#11050,10.) ;
#3122=VECTOR('',#11053,10.) ;
#3123=VECTOR('',#11054,10.) ;
#3124=VECTOR('',#11063,10.) ;
#3125=VECTOR('',#11064,10.) ;
#3126=VECTOR('',#11065,10.) ;
#3127=VECTOR('',#11066,10.) ;
#3128=VECTOR('',#11069,10.) ;
#3129=VECTOR('',#11070,10.) ;
#3130=VECTOR('',#11071,10.) ;
#3131=VECTOR('',#11074,10.) ;
#3132=VECTOR('',#11075,10.) ;
#3133=VECTOR('',#11080,3.99999999999999) ;
#3134=VECTOR('',#11097,10.) ;
#3135=VECTOR('',#11100,10.) ;
#3136=VECTOR('',#11101,10.) ;
#3137=VECTOR('',#11110,10.) ;
#3138=VECTOR('',#11111,10.) ;
#3139=VECTOR('',#11112,10.) ;
#3140=VECTOR('',#11113,10.) ;
#3141=VECTOR('',#11116,10.) ;
#3142=VECTOR('',#11117,10.) ;
#3143=VECTOR('',#11118,10.) ;
#3144=VECTOR('',#11121,10.) ;
#3145=VECTOR('',#11122,10.) ;
#3146=VECTOR('',#11125,10.) ;
#3147=VECTOR('',#11126,10.) ;
#3148=VECTOR('',#11127,10.) ;
#3149=VECTOR('',#11130,10.) ;
#3150=VECTOR('',#11131,10.) ;
#3151=VECTOR('',#11132,10.) ;
#3152=VECTOR('',#11135,10.) ;
#3153=VECTOR('',#11136,10.) ;
#3154=VECTOR('',#11139,10.) ;
#3155=VECTOR('',#11142,10.) ;
#3156=VECTOR('',#11143,10.) ;
#3157=VECTOR('',#11144,10.) ;
#3158=VECTOR('',#11147,10.) ;
#3159=VECTOR('',#11148,10.) ;
#3160=VECTOR('',#11151,10.) ;
#3161=VECTOR('',#11152,10.) ;
#3162=VECTOR('',#11155,10.) ;
#3163=VECTOR('',#11156,10.) ;
#3164=VECTOR('',#11159,10.) ;
#3165=VECTOR('',#11160,10.) ;
#3166=VECTOR('',#11161,10.) ;
#3167=VECTOR('',#11162,10.) ;
#3168=VECTOR('',#11163,10.) ;
#3169=VECTOR('',#11164,10.) ;
#3170=VECTOR('',#11167,10.) ;
#3171=VECTOR('',#11168,10.) ;
#3172=VECTOR('',#11169,10.) ;
#3173=VECTOR('',#11172,10.) ;
#3174=VECTOR('',#11173,10.) ;
#3175=VECTOR('',#11176,10.) ;
#3176=VECTOR('',#11177,10.) ;
#3177=VECTOR('',#11180,10.) ;
#3178=VECTOR('',#11181,10.) ;
#3179=VECTOR('',#11182,10.) ;
#3180=VECTOR('',#11185,10.) ;
#3181=VECTOR('',#11188,10.) ;
#3182=VECTOR('',#11191,10.) ;
#3183=VECTOR('',#11194,10.) ;
#3184=VECTOR('',#11197,10.) ;
#3185=VECTOR('',#11198,10.) ;
#3186=VECTOR('',#11201,10.) ;
#3187=VECTOR('',#11202,10.) ;
#3188=VECTOR('',#11205,10.) ;
#3189=VECTOR('',#11208,10.) ;
#3190=VECTOR('',#11213,10.) ;
#3191=VECTOR('',#11216,10.) ;
#3775=CIRCLE('',#9750,1.20000000000001) ;
#3776=CIRCLE('',#9751,1.05) ;
#3777=CIRCLE('',#9753,1.2) ;
#3778=CIRCLE('',#9755,1.05) ;
#3779=CIRCLE('',#9757,1.20000000000001) ;
#3780=CIRCLE('',#9758,1.05) ;
#3781=CIRCLE('',#9760,1.2) ;
#3782=CIRCLE('',#9762,1.05) ;
#3783=CIRCLE('',#9764,1.20000000000001) ;
#3784=CIRCLE('',#9765,1.05) ;
#3785=CIRCLE('',#9767,1.2) ;
#3786=CIRCLE('',#9769,1.05) ;
#3787=CIRCLE('',#9771,1.20000000000001) ;
#3788=CIRCLE('',#9772,1.05) ;
#3789=CIRCLE('',#9774,1.2) ;
#3790=CIRCLE('',#9776,1.05) ;
#3791=CIRCLE('',#9778,1.05) ;
#3792=CIRCLE('',#9780,1.05) ;
#3793=CIRCLE('',#9781,1.05) ;
#3794=CIRCLE('',#9783,1.05) ;
#3795=CIRCLE('',#9785,1.05) ;
#3796=CIRCLE('',#9786,1.05) ;
#3797=CIRCLE('',#9788,1.05) ;
#3798=CIRCLE('',#9790,1.05) ;
#3799=CIRCLE('',#9792,1.05) ;
#3800=CIRCLE('',#9794,1.05) ;
#3801=CIRCLE('',#9801,2.05) ;
#3802=CIRCLE('',#9802,2.05) ;
#3803=CIRCLE('',#9806,2.05) ;
#3804=CIRCLE('',#9807,2.05) ;
#3805=CIRCLE('',#9811,2.95) ;
#3806=CIRCLE('',#9812,2.95) ;
#3807=CIRCLE('',#9816,2.95) ;
#3808=CIRCLE('',#9817,2.95) ;
#3809=CIRCLE('',#9820,2.05) ;
#3810=CIRCLE('',#9821,2.05) ;
#3811=CIRCLE('',#9823,2.05) ;
#3812=CIRCLE('',#9824,2.05) ;
#3813=CIRCLE('',#9826,2.05) ;
#3814=CIRCLE('',#9827,2.05) ;
#3815=CIRCLE('',#9829,2.05) ;
#3816=CIRCLE('',#9830,2.05) ;
#3817=CIRCLE('',#9833,3.50000000000001) ;
#3818=CIRCLE('',#9836,3.50000000000001) ;
#3819=CIRCLE('',#9843,3.99999999999999) ;
#3820=CIRCLE('',#9844,3.99999999999999) ;
#3821=CIRCLE('',#9845,3.99999999999999) ;
#3822=CIRCLE('',#9846,3.99999999999999) ;
#3823=CIRCLE('',#9847,3.99999999999999) ;
#3824=CIRCLE('',#9848,3.99999999999999) ;
#3825=CIRCLE('',#9854,3.99999999999999) ;
#3826=CIRCLE('',#9858,3.50000000000001) ;
#3827=CIRCLE('',#9864,3.99999999999999) ;
#3828=CIRCLE('',#9865,3.99999999999999) ;
#3829=CIRCLE('',#9866,3.99999999999999) ;
#3830=CIRCLE('',#9867,3.99999999999999) ;
#3831=CIRCLE('',#9868,3.99999999999999) ;
#3832=CIRCLE('',#9875,3.50000000000001) ;
#4150=VERTEX_POINT('',#13425) ;
#4151=VERTEX_POINT('',#13427) ;
#4152=VERTEX_POINT('',#13431) ;
#4153=VERTEX_POINT('',#13432) ;
#4154=VERTEX_POINT('',#13434) ;
#4155=VERTEX_POINT('',#13436) ;
#4156=VERTEX_POINT('',#13439) ;
#4157=VERTEX_POINT('',#13442) ;
#4158=VERTEX_POINT('',#13446) ;
#4159=VERTEX_POINT('',#13448) ;
#4160=VERTEX_POINT('',#13452) ;
#4161=VERTEX_POINT('',#13453) ;
#4162=VERTEX_POINT('',#13455) ;
#4163=VERTEX_POINT('',#13457) ;
#4164=VERTEX_POINT('',#13460) ;
#4165=VERTEX_POINT('',#13463) ;
#4166=VERTEX_POINT('',#13467) ;
#4167=VERTEX_POINT('',#13469) ;
#4168=VERTEX_POINT('',#13473) ;
#4169=VERTEX_POINT('',#13474) ;
#4170=VERTEX_POINT('',#13476) ;
#4171=VERTEX_POINT('',#13478) ;
#4172=VERTEX_POINT('',#13481) ;
#4173=VERTEX_POINT('',#13484) ;
#4174=VERTEX_POINT('',#13488) ;
#4175=VERTEX_POINT('',#13490) ;
#4176=VERTEX_POINT('',#13494) ;
#4177=VERTEX_POINT('',#13495) ;
#4178=VERTEX_POINT('',#13497) ;
#4179=VERTEX_POINT('',#13499) ;
#4180=VERTEX_POINT('',#13502) ;
#4181=VERTEX_POINT('',#13505) ;
#4182=VERTEX_POINT('',#13509) ;
#4183=VERTEX_POINT('',#13513) ;
#4184=VERTEX_POINT('',#13515) ;
#4185=VERTEX_POINT('',#13517) ;
#4186=VERTEX_POINT('',#13555) ;
#4187=VERTEX_POINT('',#13559) ;
#4188=VERTEX_POINT('',#13561) ;
#4189=VERTEX_POINT('',#13563) ;
#4190=VERTEX_POINT('',#13601) ;
#4191=VERTEX_POINT('',#13605) ;
#4192=VERTEX_POINT('',#13609) ;
#4193=VERTEX_POINT('',#13613) ;
#4194=VERTEX_POINT('',#13617) ;
#4195=VERTEX_POINT('',#13620) ;
#4196=VERTEX_POINT('',#13623) ;
#4197=VERTEX_POINT('',#13626) ;
#4198=VERTEX_POINT('',#13637) ;
#4199=VERTEX_POINT('',#13639) ;
#4200=VERTEX_POINT('',#13643) ;
#4201=VERTEX_POINT('',#13654) ;
#4202=VERTEX_POINT('',#13656) ;
#4203=VERTEX_POINT('',#13660) ;
#4204=VERTEX_POINT('',#13663) ;
#4205=VERTEX_POINT('',#13664) ;
#4206=VERTEX_POINT('',#13701) ;
#4207=VERTEX_POINT('',#13703) ;
#4208=VERTEX_POINT('',#13741) ;
#4209=VERTEX_POINT('',#13743) ;
#4210=VERTEX_POINT('',#13748) ;
#4211=VERTEX_POINT('',#13749) ;
#4212=VERTEX_POINT('',#13786) ;
#4213=VERTEX_POINT('',#13788) ;
#4214=VERTEX_POINT('',#13826) ;
#4215=VERTEX_POINT('',#13828) ;
#4216=VERTEX_POINT('',#13833) ;
#4217=VERTEX_POINT('',#13835) ;
#4218=VERTEX_POINT('',#13839) ;
#4219=VERTEX_POINT('',#13841) ;
#4220=VERTEX_POINT('',#13845) ;
#4221=VERTEX_POINT('',#13846) ;
#4222=VERTEX_POINT('',#13848) ;
#4223=VERTEX_POINT('',#13850) ;
#4224=VERTEX_POINT('',#13854) ;
#4225=VERTEX_POINT('',#13855) ;
#4226=VERTEX_POINT('',#13857) ;
#4227=VERTEX_POINT('',#13859) ;
#4228=VERTEX_POINT('',#13863) ;
#4229=VERTEX_POINT('',#13865) ;
#4230=VERTEX_POINT('',#13869) ;
#4231=VERTEX_POINT('',#13871) ;
#4232=VERTEX_POINT('',#13873) ;
#4233=VERTEX_POINT('',#13877) ;
#4234=VERTEX_POINT('',#13879) ;
#4235=VERTEX_POINT('',#13883) ;
#4236=VERTEX_POINT('',#13885) ;
#4237=VERTEX_POINT('',#13887) ;
#4238=VERTEX_POINT('',#13891) ;
#4239=VERTEX_POINT('',#13892) ;
#4240=VERTEX_POINT('',#13894) ;
#4241=VERTEX_POINT('',#13896) ;
#4242=VERTEX_POINT('',#13900) ;
#4243=VERTEX_POINT('',#13902) ;
#4244=VERTEX_POINT('',#13904) ;
#4245=VERTEX_POINT('',#13906) ;
#4246=VERTEX_POINT('',#13910) ;
#4247=VERTEX_POINT('',#13912) ;
#4248=VERTEX_POINT('',#13914) ;
#4249=VERTEX_POINT('',#13916) ;
#4250=VERTEX_POINT('',#13918) ;
#4251=VERTEX_POINT('',#13920) ;
#4252=VERTEX_POINT('',#13922) ;
#4253=VERTEX_POINT('',#13924) ;
#4254=VERTEX_POINT('',#13926) ;
#4255=VERTEX_POINT('',#13928) ;
#4256=VERTEX_POINT('',#13930) ;
#4257=VERTEX_POINT('',#13932) ;
#4258=VERTEX_POINT('',#13935) ;
#4259=VERTEX_POINT('',#13937) ;
#4260=VERTEX_POINT('',#13940) ;
#4261=VERTEX_POINT('',#13944) ;
#4262=VERTEX_POINT('',#13946) ;
#4263=VERTEX_POINT('',#13950) ;
#4264=VERTEX_POINT('',#13952) ;
#4265=VERTEX_POINT('',#13954) ;
#4266=VERTEX_POINT('',#13958) ;
#4267=VERTEX_POINT('',#13960) ;
#4268=VERTEX_POINT('',#13962) ;
#4269=VERTEX_POINT('',#13964) ;
#4270=VERTEX_POINT('',#13968) ;
#4271=VERTEX_POINT('',#13970) ;
#4272=VERTEX_POINT('',#13978) ;
#4273=VERTEX_POINT('',#13980) ;
#4274=VERTEX_POINT('',#13982) ;
#4275=VERTEX_POINT('',#13984) ;
#4276=VERTEX_POINT('',#13986) ;
#4277=VERTEX_POINT('',#13988) ;
#4278=VERTEX_POINT('',#13990) ;
#4279=VERTEX_POINT('',#13992) ;
#4280=VERTEX_POINT('',#13994) ;
#4281=VERTEX_POINT('',#13996) ;
#4282=VERTEX_POINT('',#13999) ;
#4283=VERTEX_POINT('',#14001) ;
#4284=VERTEX_POINT('',#14004) ;
#4285=VERTEX_POINT('',#14006) ;
#4286=VERTEX_POINT('',#14014) ;
#4287=VERTEX_POINT('',#14021) ;
#4288=VERTEX_POINT('',#14022) ;
#4289=VERTEX_POINT('',#14024) ;
#4290=VERTEX_POINT('',#14026) ;
#4291=VERTEX_POINT('',#14030) ;
#4292=VERTEX_POINT('',#14032) ;
#4293=VERTEX_POINT('',#14036) ;
#4294=VERTEX_POINT('',#14040) ;
#4295=VERTEX_POINT('',#14042) ;
#4296=VERTEX_POINT('',#14054) ;
#4297=VERTEX_POINT('',#14061) ;
#4298=VERTEX_POINT('',#14062) ;
#4299=VERTEX_POINT('',#14064) ;
#4300=VERTEX_POINT('',#14066) ;
#4301=VERTEX_POINT('',#14070) ;
#4302=VERTEX_POINT('',#14072) ;
#4303=VERTEX_POINT('',#14076) ;
#4304=VERTEX_POINT('',#14080) ;
#4305=VERTEX_POINT('',#14082) ;
#4306=VERTEX_POINT('',#14086) ;
#4307=VERTEX_POINT('',#14088) ;
#4308=VERTEX_POINT('',#14097) ;
#4309=VERTEX_POINT('',#14099) ;
#4310=VERTEX_POINT('',#14106) ;
#4311=VERTEX_POINT('',#14110) ;
#4312=VERTEX_POINT('',#14115) ;
#4313=VERTEX_POINT('',#14119) ;
#4314=VERTEX_POINT('',#14123) ;
#4315=VERTEX_POINT('',#14125) ;
#4316=VERTEX_POINT('',#14132) ;
#4317=VERTEX_POINT('',#14136) ;
#4318=VERTEX_POINT('',#14149) ;
#4319=VERTEX_POINT('',#14153) ;
#5018=EDGE_CURVE('',#4150,#4150,#3775,.T.) ;
#5019=EDGE_CURVE('',#4150,#4151,#2233,.T.) ;
#5020=EDGE_CURVE('',#4151,#4151,#3776,.T.) ;
#5021=EDGE_CURVE('',#4152,#4153,#2234,.T.) ;
#5022=EDGE_CURVE('',#4154,#4152,#2235,.T.) ;
#5023=EDGE_CURVE('',#4155,#4154,#2236,.T.) ;
#5024=EDGE_CURVE('',#4153,#4155,#2237,.T.) ;
#5025=EDGE_CURVE('',#4156,#4156,#3777,.T.) ;
#5026=EDGE_CURVE('',#4151,#4157,#2238,.T.) ;
#5027=EDGE_CURVE('',#4157,#4157,#3778,.T.) ;
#5028=EDGE_CURVE('',#4158,#4158,#3779,.T.) ;
#5029=EDGE_CURVE('',#4158,#4159,#2239,.T.) ;
#5030=EDGE_CURVE('',#4159,#4159,#3780,.T.) ;
#5031=EDGE_CURVE('',#4160,#4161,#2240,.T.) ;
#5032=EDGE_CURVE('',#4162,#4160,#2241,.T.) ;
#5033=EDGE_CURVE('',#4163,#4162,#2242,.T.) ;
#5034=EDGE_CURVE('',#4161,#4163,#2243,.T.) ;
#5035=EDGE_CURVE('',#4164,#4164,#3781,.T.) ;
#5036=EDGE_CURVE('',#4159,#4165,#2244,.T.) ;
#5037=EDGE_CURVE('',#4165,#4165,#3782,.T.) ;
#5038=EDGE_CURVE('',#4166,#4166,#3783,.T.) ;
#5039=EDGE_CURVE('',#4166,#4167,#2245,.T.) ;
#5040=EDGE_CURVE('',#4167,#4167,#3784,.T.) ;
#5041=EDGE_CURVE('',#4168,#4169,#2246,.T.) ;
#5042=EDGE_CURVE('',#4170,#4168,#2247,.T.) ;
#5043=EDGE_CURVE('',#4171,#4170,#2248,.T.) ;
#5044=EDGE_CURVE('',#4169,#4171,#2249,.T.) ;
#5045=EDGE_CURVE('',#4172,#4172,#3785,.T.) ;
#5046=EDGE_CURVE('',#4167,#4173,#2250,.T.) ;
#5047=EDGE_CURVE('',#4173,#4173,#3786,.T.) ;
#5048=EDGE_CURVE('',#4174,#4174,#3787,.T.) ;
#5049=EDGE_CURVE('',#4174,#4175,#2251,.T.) ;
#5050=EDGE_CURVE('',#4175,#4175,#3788,.T.) ;
#5051=EDGE_CURVE('',#4176,#4177,#2252,.T.) ;
#5052=EDGE_CURVE('',#4178,#4176,#2253,.T.) ;
#5053=EDGE_CURVE('',#4179,#4178,#2254,.T.) ;
#5054=EDGE_CURVE('',#4177,#4179,#2255,.T.) ;
#5055=EDGE_CURVE('',#4180,#4180,#3789,.T.) ;
#5056=EDGE_CURVE('',#4175,#4181,#2256,.T.) ;
#5057=EDGE_CURVE('',#4181,#4181,#3790,.T.) ;
#5058=EDGE_CURVE('',#4172,#4182,#2257,.T.) ;
#5059=EDGE_CURVE('',#4182,#4182,#3791,.T.) ;
#5060=EDGE_CURVE('',#4182,#4183,#2258,.T.) ;
#5061=EDGE_CURVE('',#4183,#4184,#3792,.T.) ;
#5062=EDGE_CURVE('',#4185,#4184,#407,.T.) ;
#5063=EDGE_CURVE('',#4185,#4183,#3793,.T.) ;
#5064=EDGE_CURVE('',#4180,#4186,#2259,.T.) ;
#5065=EDGE_CURVE('',#4186,#4186,#3794,.T.) ;
#5066=EDGE_CURVE('',#4186,#4187,#2260,.T.) ;
#5067=EDGE_CURVE('',#4187,#4188,#3795,.T.) ;
#5068=EDGE_CURVE('',#4189,#4188,#408,.T.) ;
#5069=EDGE_CURVE('',#4189,#4187,#3796,.T.) ;
#5070=EDGE_CURVE('',#4164,#4190,#2261,.T.) ;
#5071=EDGE_CURVE('',#4190,#4190,#3797,.T.) ;
#5072=EDGE_CURVE('',#4190,#4191,#2262,.T.) ;
#5073=EDGE_CURVE('',#4191,#4191,#3798,.T.) ;
#5074=EDGE_CURVE('',#4156,#4192,#2263,.T.) ;
#5075=EDGE_CURVE('',#4192,#4192,#3799,.T.) ;
#5076=EDGE_CURVE('',#4192,#4193,#2264,.T.) ;
#5077=EDGE_CURVE('',#4193,#4193,#3800,.T.) ;
#5078=EDGE_CURVE('',#4157,#4194,#2265,.T.) ;
#5079=EDGE_CURVE('',#4193,#4195,#2266,.T.) ;
#5080=EDGE_CURVE('',#4165,#4196,#2267,.T.) ;
#5081=EDGE_CURVE('',#4191,#4197,#2268,.T.) ;
#5082=EDGE_CURVE('',#4188,#4189,#409,.T.) ;
#5083=EDGE_CURVE('',#4198,#4198,#3801,.T.) ;
#5084=EDGE_CURVE('',#4198,#4199,#2269,.T.) ;
#5085=EDGE_CURVE('',#4199,#4199,#3802,.T.) ;
#5086=EDGE_CURVE('',#4181,#4200,#2270,.T.) ;
#5087=EDGE_CURVE('',#4184,#4185,#410,.T.) ;
#5088=EDGE_CURVE('',#4201,#4201,#3803,.T.) ;
#5089=EDGE_CURVE('',#4201,#4202,#2271,.T.) ;
#5090=EDGE_CURVE('',#4202,#4202,#3804,.T.) ;
#5091=EDGE_CURVE('',#4173,#4203,#2272,.T.) ;
#5092=EDGE_CURVE('',#4204,#4205,#411,.T.) ;
#5093=EDGE_CURVE('',#4205,#4204,#412,.T.) ;
#5094=EDGE_CURVE('',#4205,#4206,#2273,.T.) ;
#5095=EDGE_CURVE('',#4207,#4206,#413,.T.) ;
#5096=EDGE_CURVE('',#4206,#4207,#414,.T.) ;
#5097=EDGE_CURVE('',#4208,#4208,#3805,.T.) ;
#5098=EDGE_CURVE('',#4208,#4209,#2274,.T.) ;
#5099=EDGE_CURVE('',#4209,#4209,#3806,.T.) ;
#5100=EDGE_CURVE('',#4210,#4211,#415,.T.) ;
#5101=EDGE_CURVE('',#4211,#4210,#416,.T.) ;
#5102=EDGE_CURVE('',#4211,#4212,#2275,.T.) ;
#5103=EDGE_CURVE('',#4213,#4212,#417,.T.) ;
#5104=EDGE_CURVE('',#4212,#4213,#418,.T.) ;
#5105=EDGE_CURVE('',#4214,#4214,#3807,.T.) ;
#5106=EDGE_CURVE('',#4214,#4215,#2276,.T.) ;
#5107=EDGE_CURVE('',#4215,#4215,#3808,.T.) ;
#5108=EDGE_CURVE('',#4216,#4216,#3809,.T.) ;
#5109=EDGE_CURVE('',#4216,#4217,#2277,.T.) ;
#5110=EDGE_CURVE('',#4217,#4217,#3810,.T.) ;
#5111=EDGE_CURVE('',#4218,#4218,#3811,.T.) ;
#5112=EDGE_CURVE('',#4218,#4219,#2278,.T.) ;
#5113=EDGE_CURVE('',#4219,#4219,#3812,.T.) ;
#5114=EDGE_CURVE('',#4220,#4221,#2279,.T.) ;
#5115=EDGE_CURVE('',#4222,#4220,#3813,.T.) ;
#5116=EDGE_CURVE('',#4223,#4222,#2280,.T.) ;
#5117=EDGE_CURVE('',#4221,#4223,#3814,.T.) ;
#5118=EDGE_CURVE('',#4224,#4225,#2281,.T.) ;
#5119=EDGE_CURVE('',#4226,#4224,#3815,.T.) ;
#5120=EDGE_CURVE('',#4227,#4226,#2282,.T.) ;
#5121=EDGE_CURVE('',#4225,#4227,#3816,.T.) ;
#5122=EDGE_CURVE('',#4228,#4226,#2283,.T.) ;
#5123=EDGE_CURVE('',#4229,#4228,#2284,.T.) ;
#5124=EDGE_CURVE('',#4229,#4227,#2285,.T.) ;
#5125=EDGE_CURVE('',#4224,#4230,#3817,.T.) ;
#5126=EDGE_CURVE('',#4230,#4231,#2286,.T.) ;
#5127=EDGE_CURVE('',#4232,#4231,#2287,.T.) ;
#5128=EDGE_CURVE('',#4232,#4228,#2288,.T.) ;
#5129=EDGE_CURVE('',#4233,#4222,#2289,.T.) ;
#5130=EDGE_CURVE('',#4234,#4233,#2290,.T.) ;
#5131=EDGE_CURVE('',#4234,#4223,#2291,.T.) ;
#5132=EDGE_CURVE('',#4220,#4235,#3818,.T.) ;
#5133=EDGE_CURVE('',#4235,#4236,#2292,.T.) ;
#5134=EDGE_CURVE('',#4237,#4236,#2293,.T.) ;
#5135=EDGE_CURVE('',#4237,#4233,#2294,.T.) ;
#5136=EDGE_CURVE('',#4238,#4239,#2295,.T.) ;
#5137=EDGE_CURVE('',#4239,#4240,#2296,.T.) ;
#5138=EDGE_CURVE('',#4240,#4241,#2297,.T.) ;
#5139=EDGE_CURVE('',#4241,#4238,#2298,.T.) ;
#5140=EDGE_CURVE('',#4242,#4241,#2299,.T.) ;
#5141=EDGE_CURVE('',#4242,#4243,#2300,.T.) ;
#5142=EDGE_CURVE('',#4243,#4244,#2301,.T.) ;
#5143=EDGE_CURVE('',#4244,#4245,#2302,.T.) ;
#5144=EDGE_CURVE('',#4245,#4238,#2303,.T.) ;
#5145=EDGE_CURVE('',#4246,#4240,#2304,.T.) ;
#5146=EDGE_CURVE('',#4246,#4247,#2305,.T.) ;
#5147=EDGE_CURVE('',#4247,#4248,#2306,.T.) ;
#5148=EDGE_CURVE('',#4248,#4249,#2307,.T.) ;
#5149=EDGE_CURVE('',#4250,#4249,#2308,.T.) ;
#5150=EDGE_CURVE('',#4250,#4251,#2309,.T.) ;
#5151=EDGE_CURVE('',#4251,#4252,#2310,.T.) ;
#5152=EDGE_CURVE('',#4252,#4253,#2311,.T.) ;
#5153=EDGE_CURVE('',#4254,#4253,#2312,.T.) ;
#5154=EDGE_CURVE('',#4255,#4254,#2313,.T.) ;
#5155=EDGE_CURVE('',#4256,#4255,#2314,.T.) ;
#5156=EDGE_CURVE('',#4257,#4256,#2315,.T.) ;
#5157=EDGE_CURVE('',#4179,#4257,#2316,.T.) ;
#5158=EDGE_CURVE('',#4178,#4258,#2317,.T.) ;
#5159=EDGE_CURVE('',#4258,#4259,#2318,.T.) ;
#5160=EDGE_CURVE('',#4171,#4259,#2319,.T.) ;
#5161=EDGE_CURVE('',#4170,#4260,#2320,.T.) ;
#5162=EDGE_CURVE('',#4242,#4260,#2321,.T.) ;
#5163=EDGE_CURVE('',#4254,#4261,#2322,.T.) ;
#5164=EDGE_CURVE('',#4261,#4262,#2323,.T.) ;
#5165=EDGE_CURVE('',#4262,#4255,#2324,.T.) ;
#5166=EDGE_CURVE('',#4263,#4262,#2325,.T.) ;
#5167=EDGE_CURVE('',#4263,#4264,#2326,.T.) ;
#5168=EDGE_CURVE('',#4264,#4265,#2327,.T.) ;
#5169=EDGE_CURVE('',#4265,#4256,#2328,.T.) ;
#5170=EDGE_CURVE('',#4266,#4266,#3819,.T.) ;
#5171=EDGE_CURVE('',#4266,#4267,#2329,.T.) ;
#5172=EDGE_CURVE('',#4267,#4268,#3820,.T.) ;
#5173=EDGE_CURVE('',#4269,#4268,#2330,.T.) ;
#5174=EDGE_CURVE('',#4253,#4269,#3821,.T.) ;
#5175=EDGE_CURVE('',#4252,#4251,#3822,.T.) ;
#5176=EDGE_CURVE('',#4270,#4250,#3823,.T.) ;
#5177=EDGE_CURVE('',#4271,#4270,#2331,.T.) ;
#5178=EDGE_CURVE('',#4271,#4267,#3824,.T.) ;
#5179=EDGE_CURVE('',#4268,#4271,#2332,.T.) ;
#5180=EDGE_CURVE('',#4272,#4270,#2333,.T.) ;
#5181=EDGE_CURVE('',#4272,#4273,#2334,.T.) ;
#5182=EDGE_CURVE('',#4273,#4274,#2335,.T.) ;
#5183=EDGE_CURVE('',#4274,#4275,#2336,.T.) ;
#5184=EDGE_CURVE('',#4276,#4275,#2337,.T.) ;
#5185=EDGE_CURVE('',#4277,#4276,#2338,.T.) ;
#5186=EDGE_CURVE('',#4277,#4278,#2339,.T.) ;
#5187=EDGE_CURVE('',#4278,#4279,#2340,.T.) ;
#5188=EDGE_CURVE('',#4279,#4280,#2341,.T.) ;
#5189=EDGE_CURVE('',#4281,#4280,#2342,.T.) ;
#5190=EDGE_CURVE('',#4269,#4281,#2343,.T.) ;
#5191=EDGE_CURVE('',#4236,#4282,#2344,.T.) ;
#5192=EDGE_CURVE('',#4282,#4283,#2345,.T.) ;
#5193=EDGE_CURVE('',#4283,#4237,#2346,.T.) ;
#5194=EDGE_CURVE('',#4231,#4284,#2347,.T.) ;
#5195=EDGE_CURVE('',#4284,#4285,#2348,.T.) ;
#5196=EDGE_CURVE('',#4285,#4232,#2349,.T.) ;
#5197=EDGE_CURVE('',#4249,#4272,#3825,.T.) ;
#5198=EDGE_CURVE('',#4285,#4229,#2350,.T.) ;
#5199=EDGE_CURVE('',#4286,#4284,#2351,.T.) ;
#5200=EDGE_CURVE('',#4286,#4230,#2352,.T.) ;
#5201=EDGE_CURVE('',#4225,#4286,#3826,.T.) ;
#5202=EDGE_CURVE('',#4287,#4288,#2353,.T.) ;
#5203=EDGE_CURVE('',#4289,#4287,#2354,.T.) ;
#5204=EDGE_CURVE('',#4289,#4290,#2355,.T.) ;
#5205=EDGE_CURVE('',#4290,#4288,#2356,.T.) ;
#5206=EDGE_CURVE('',#4288,#4291,#2357,.T.) ;
#5207=EDGE_CURVE('',#4292,#4290,#2358,.T.) ;
#5208=EDGE_CURVE('',#4292,#4291,#2359,.T.) ;
#5209=EDGE_CURVE('',#4293,#4292,#2360,.T.) ;
#5210=EDGE_CURVE('',#4293,#4289,#2361,.T.) ;
#5211=EDGE_CURVE('',#4294,#4294,#3827,.T.) ;
#5212=EDGE_CURVE('',#4294,#4295,#2362,.T.) ;
#5213=EDGE_CURVE('',#4295,#4273,#3828,.T.) ;
#5214=EDGE_CURVE('',#4248,#4247,#3829,.T.) ;
#5215=EDGE_CURVE('',#4275,#4246,#3830,.T.) ;
#5216=EDGE_CURVE('',#4274,#4295,#3831,.T.) ;
#5217=EDGE_CURVE('',#4283,#4234,#2363,.T.) ;
#5218=EDGE_CURVE('',#4296,#4282,#2364,.T.) ;
#5219=EDGE_CURVE('',#4296,#4235,#2365,.T.) ;
#5220=EDGE_CURVE('',#4221,#4296,#3832,.T.) ;
#5221=EDGE_CURVE('',#4297,#4298,#2366,.T.) ;
#5222=EDGE_CURVE('',#4297,#4299,#2367,.T.) ;
#5223=EDGE_CURVE('',#4299,#4300,#2368,.T.) ;
#5224=EDGE_CURVE('',#4298,#4300,#2369,.T.) ;
#5225=EDGE_CURVE('',#4301,#4297,#2370,.T.) ;
#5226=EDGE_CURVE('',#4301,#4302,#2371,.T.) ;
#5227=EDGE_CURVE('',#4302,#4299,#2372,.T.) ;
#5228=EDGE_CURVE('',#4302,#4303,#2373,.T.) ;
#5229=EDGE_CURVE('',#4300,#4303,#2374,.T.) ;
#5230=EDGE_CURVE('',#4263,#4304,#2375,.T.) ;
#5231=EDGE_CURVE('',#4304,#4305,#2376,.T.) ;
#5232=EDGE_CURVE('',#4305,#4264,#2377,.T.) ;
#5233=EDGE_CURVE('',#4152,#4306,#2378,.T.) ;
#5234=EDGE_CURVE('',#4307,#4306,#2379,.T.) ;
#5235=EDGE_CURVE('',#4154,#4307,#2380,.T.) ;
#5236=EDGE_CURVE('',#4264,#4307,#2381,.T.) ;
#5237=EDGE_CURVE('',#4155,#4305,#2382,.T.) ;
#5238=EDGE_CURVE('',#4153,#4304,#2383,.T.) ;
#5239=EDGE_CURVE('',#4244,#4308,#2384,.T.) ;
#5240=EDGE_CURVE('',#4308,#4309,#2385,.T.) ;
#5241=EDGE_CURVE('',#4309,#4245,#2386,.T.) ;
#5242=EDGE_CURVE('',#4160,#4309,#2387,.T.) ;
#5243=EDGE_CURVE('',#4162,#4308,#2388,.T.) ;
#5244=EDGE_CURVE('',#4310,#4244,#2389,.T.) ;
#5245=EDGE_CURVE('',#4163,#4310,#2390,.T.) ;
#5246=EDGE_CURVE('',#4311,#4310,#2391,.T.) ;
#5247=EDGE_CURVE('',#4161,#4311,#2392,.T.) ;
#5248=EDGE_CURVE('',#4311,#4306,#2393,.T.) ;
#5249=EDGE_CURVE('',#4243,#4312,#2394,.T.) ;
#5250=EDGE_CURVE('',#4303,#4312,#2395,.T.) ;
#5251=EDGE_CURVE('',#4291,#4301,#2396,.T.) ;
#5252=EDGE_CURVE('',#4313,#4293,#2397,.T.) ;
#5253=EDGE_CURVE('',#4313,#4265,#2398,.T.) ;
#5254=EDGE_CURVE('',#4314,#4298,#2399,.T.) ;
#5255=EDGE_CURVE('',#4315,#4314,#2400,.T.) ;
#5256=EDGE_CURVE('',#4287,#4315,#2401,.T.) ;
#5257=EDGE_CURVE('',#4312,#4277,#2402,.T.) ;
#5258=EDGE_CURVE('',#4314,#4276,#2403,.T.) ;
#5259=EDGE_CURVE('',#4265,#4316,#2404,.T.) ;
#5260=EDGE_CURVE('',#4316,#4257,#2405,.T.) ;
#5261=EDGE_CURVE('',#4176,#4317,#2406,.T.) ;
#5262=EDGE_CURVE('',#4279,#4317,#2407,.T.) ;
#5263=EDGE_CURVE('',#4258,#4279,#2408,.T.) ;
#5264=EDGE_CURVE('',#4177,#4316,#2409,.T.) ;
#5265=EDGE_CURVE('',#4317,#4313,#2410,.T.) ;
#5266=EDGE_CURVE('',#4280,#4313,#2411,.T.) ;
#5267=EDGE_CURVE('',#4278,#4259,#2412,.T.) ;
#5268=EDGE_CURVE('',#4260,#4318,#2413,.T.) ;
#5269=EDGE_CURVE('',#4318,#4243,#2414,.T.) ;
#5270=EDGE_CURVE('',#4312,#4319,#2415,.T.) ;
#5271=EDGE_CURVE('',#4319,#4278,#2416,.T.) ;
#5272=EDGE_CURVE('',#4168,#4318,#2417,.T.) ;
#5273=EDGE_CURVE('',#4169,#4319,#2418,.T.) ;
#5274=EDGE_CURVE('',#4281,#4315,#2419,.T.) ;
#5275=EDGE_CURVE('',#4239,#4261,#2420,.T.) ;
#6343=ORIENTED_EDGE('',*,*,#5018,.T.) ;
#6344=ORIENTED_EDGE('',*,*,#5019,.T.) ;
#6345=ORIENTED_EDGE('',*,*,#5020,.T.) ;
#6346=ORIENTED_EDGE('',*,*,#5019,.F.) ;
#6347=ORIENTED_EDGE('',*,*,#5021,.F.) ;
#6348=ORIENTED_EDGE('',*,*,#5022,.F.) ;
#6349=ORIENTED_EDGE('',*,*,#5023,.F.) ;
#6350=ORIENTED_EDGE('',*,*,#5024,.F.) ;
#6351=ORIENTED_EDGE('',*,*,#5025,.F.) ;
#6352=ORIENTED_EDGE('',*,*,#5018,.F.) ;
#6353=ORIENTED_EDGE('',*,*,#5020,.F.) ;
#6354=ORIENTED_EDGE('',*,*,#5026,.T.) ;
#6355=ORIENTED_EDGE('',*,*,#5027,.T.) ;
#6356=ORIENTED_EDGE('',*,*,#5026,.F.) ;
#6357=ORIENTED_EDGE('',*,*,#5028,.T.) ;
#6358=ORIENTED_EDGE('',*,*,#5029,.T.) ;
#6359=ORIENTED_EDGE('',*,*,#5030,.T.) ;
#6360=ORIENTED_EDGE('',*,*,#5029,.F.) ;
#6361=ORIENTED_EDGE('',*,*,#5031,.F.) ;
#6362=ORIENTED_EDGE('',*,*,#5032,.F.) ;
#6363=ORIENTED_EDGE('',*,*,#5033,.F.) ;
#6364=ORIENTED_EDGE('',*,*,#5034,.F.) ;
#6365=ORIENTED_EDGE('',*,*,#5035,.F.) ;
#6366=ORIENTED_EDGE('',*,*,#5028,.F.) ;
#6367=ORIENTED_EDGE('',*,*,#5030,.F.) ;
#6368=ORIENTED_EDGE('',*,*,#5036,.T.) ;
#6369=ORIENTED_EDGE('',*,*,#5037,.T.) ;
#6370=ORIENTED_EDGE('',*,*,#5036,.F.) ;
#6371=ORIENTED_EDGE('',*,*,#5038,.T.) ;
#6372=ORIENTED_EDGE('',*,*,#5039,.T.) ;
#6373=ORIENTED_EDGE('',*,*,#5040,.T.) ;
#6374=ORIENTED_EDGE('',*,*,#5039,.F.) ;
#6375=ORIENTED_EDGE('',*,*,#5041,.F.) ;
#6376=ORIENTED_EDGE('',*,*,#5042,.F.) ;
#6377=ORIENTED_EDGE('',*,*,#5043,.F.) ;
#6378=ORIENTED_EDGE('',*,*,#5044,.F.) ;
#6379=ORIENTED_EDGE('',*,*,#5045,.F.) ;
#6380=ORIENTED_EDGE('',*,*,#5038,.F.) ;
#6381=ORIENTED_EDGE('',*,*,#5040,.F.) ;
#6382=ORIENTED_EDGE('',*,*,#5046,.T.) ;
#6383=ORIENTED_EDGE('',*,*,#5047,.T.) ;
#6384=ORIENTED_EDGE('',*,*,#5046,.F.) ;
#6385=ORIENTED_EDGE('',*,*,#5048,.T.) ;
#6386=ORIENTED_EDGE('',*,*,#5049,.T.) ;
#6387=ORIENTED_EDGE('',*,*,#5050,.T.) ;
#6388=ORIENTED_EDGE('',*,*,#5049,.F.) ;
#6389=ORIENTED_EDGE('',*,*,#5051,.F.) ;
#6390=ORIENTED_EDGE('',*,*,#5052,.F.) ;
#6391=ORIENTED_EDGE('',*,*,#5053,.F.) ;
#6392=ORIENTED_EDGE('',*,*,#5054,.F.) ;
#6393=ORIENTED_EDGE('',*,*,#5055,.F.) ;
#6394=ORIENTED_EDGE('',*,*,#5048,.F.) ;
#6395=ORIENTED_EDGE('',*,*,#5050,.F.) ;
#6396=ORIENTED_EDGE('',*,*,#5056,.T.) ;
#6397=ORIENTED_EDGE('',*,*,#5057,.T.) ;
#6398=ORIENTED_EDGE('',*,*,#5056,.F.) ;
#6399=ORIENTED_EDGE('',*,*,#5045,.T.) ;
#6400=ORIENTED_EDGE('',*,*,#5058,.T.) ;
#6401=ORIENTED_EDGE('',*,*,#5059,.T.) ;
#6402=ORIENTED_EDGE('',*,*,#5058,.F.) ;
#6403=ORIENTED_EDGE('',*,*,#5059,.F.) ;
#6404=ORIENTED_EDGE('',*,*,#5060,.T.) ;
#6405=ORIENTED_EDGE('',*,*,#5061,.T.) ;
#6406=ORIENTED_EDGE('',*,*,#5062,.F.) ;
#6407=ORIENTED_EDGE('',*,*,#5063,.T.) ;
#6408=ORIENTED_EDGE('',*,*,#5060,.F.) ;
#6409=ORIENTED_EDGE('',*,*,#5055,.T.) ;
#6410=ORIENTED_EDGE('',*,*,#5064,.T.) ;
#6411=ORIENTED_EDGE('',*,*,#5065,.T.) ;
#6412=ORIENTED_EDGE('',*,*,#5064,.F.) ;
#6413=ORIENTED_EDGE('',*,*,#5065,.F.) ;
#6414=ORIENTED_EDGE('',*,*,#5066,.T.) ;
#6415=ORIENTED_EDGE('',*,*,#5067,.T.) ;
#6416=ORIENTED_EDGE('',*,*,#5068,.F.) ;
#6417=ORIENTED_EDGE('',*,*,#5069,.T.) ;
#6418=ORIENTED_EDGE('',*,*,#5066,.F.) ;
#6419=ORIENTED_EDGE('',*,*,#5035,.T.) ;
#6420=ORIENTED_EDGE('',*,*,#5070,.T.) ;
#6421=ORIENTED_EDGE('',*,*,#5071,.T.) ;
#6422=ORIENTED_EDGE('',*,*,#5070,.F.) ;
#6423=ORIENTED_EDGE('',*,*,#5071,.F.) ;
#6424=ORIENTED_EDGE('',*,*,#5072,.T.) ;
#6425=ORIENTED_EDGE('',*,*,#5073,.T.) ;
#6426=ORIENTED_EDGE('',*,*,#5072,.F.) ;
#6427=ORIENTED_EDGE('',*,*,#5025,.T.) ;
#6428=ORIENTED_EDGE('',*,*,#5074,.T.) ;
#6429=ORIENTED_EDGE('',*,*,#5075,.T.) ;
#6430=ORIENTED_EDGE('',*,*,#5074,.F.) ;
#6431=ORIENTED_EDGE('',*,*,#5075,.F.) ;
#6432=ORIENTED_EDGE('',*,*,#5076,.T.) ;
#6433=ORIENTED_EDGE('',*,*,#5077,.T.) ;
#6434=ORIENTED_EDGE('',*,*,#5076,.F.) ;
#6435=ORIENTED_EDGE('',*,*,#5027,.F.) ;
#6436=ORIENTED_EDGE('',*,*,#5078,.T.) ;
#6437=ORIENTED_EDGE('',*,*,#5078,.F.) ;
#6438=ORIENTED_EDGE('',*,*,#5077,.F.) ;
#6439=ORIENTED_EDGE('',*,*,#5079,.T.) ;
#6440=ORIENTED_EDGE('',*,*,#5079,.F.) ;
#6441=ORIENTED_EDGE('',*,*,#5037,.F.) ;
#6442=ORIENTED_EDGE('',*,*,#5080,.T.) ;
#6443=ORIENTED_EDGE('',*,*,#5080,.F.) ;
#6444=ORIENTED_EDGE('',*,*,#5073,.F.) ;
#6445=ORIENTED_EDGE('',*,*,#5081,.T.) ;
#6446=ORIENTED_EDGE('',*,*,#5081,.F.) ;
#6447=ORIENTED_EDGE('',*,*,#5082,.F.) ;
#6448=ORIENTED_EDGE('',*,*,#5067,.F.) ;
#6449=ORIENTED_EDGE('',*,*,#5069,.F.) ;
#6450=ORIENTED_EDGE('',*,*,#5083,.F.) ;
#6451=ORIENTED_EDGE('',*,*,#5084,.T.) ;
#6452=ORIENTED_EDGE('',*,*,#5085,.F.) ;
#6453=ORIENTED_EDGE('',*,*,#5084,.F.) ;
#6454=ORIENTED_EDGE('',*,*,#5082,.T.) ;
#6455=ORIENTED_EDGE('',*,*,#5068,.T.) ;
#6456=ORIENTED_EDGE('',*,*,#5057,.F.) ;
#6457=ORIENTED_EDGE('',*,*,#5086,.T.) ;
#6458=ORIENTED_EDGE('',*,*,#5086,.F.) ;
#6459=ORIENTED_EDGE('',*,*,#5087,.F.) ;
#6460=ORIENTED_EDGE('',*,*,#5061,.F.) ;
#6461=ORIENTED_EDGE('',*,*,#5063,.F.) ;
#6462=ORIENTED_EDGE('',*,*,#5088,.F.) ;
#6463=ORIENTED_EDGE('',*,*,#5089,.T.) ;
#6464=ORIENTED_EDGE('',*,*,#5090,.F.) ;
#6465=ORIENTED_EDGE('',*,*,#5089,.F.) ;
#6466=ORIENTED_EDGE('',*,*,#5087,.T.) ;
#6467=ORIENTED_EDGE('',*,*,#5062,.T.) ;
#6468=ORIENTED_EDGE('',*,*,#5047,.F.) ;
#6469=ORIENTED_EDGE('',*,*,#5091,.T.) ;
#6470=ORIENTED_EDGE('',*,*,#5091,.F.) ;
#6471=ORIENTED_EDGE('',*,*,#5092,.F.) ;
#6472=ORIENTED_EDGE('',*,*,#5093,.F.) ;
#6473=ORIENTED_EDGE('',*,*,#5094,.T.) ;
#6474=ORIENTED_EDGE('',*,*,#5095,.F.) ;
#6475=ORIENTED_EDGE('',*,*,#5096,.F.) ;
#6476=ORIENTED_EDGE('',*,*,#5094,.F.) ;
#6477=ORIENTED_EDGE('',*,*,#5097,.F.) ;
#6478=ORIENTED_EDGE('',*,*,#5098,.T.) ;
#6479=ORIENTED_EDGE('',*,*,#5099,.T.) ;
#6480=ORIENTED_EDGE('',*,*,#5098,.F.) ;
#6481=ORIENTED_EDGE('',*,*,#5095,.T.) ;
#6482=ORIENTED_EDGE('',*,*,#5096,.T.) ;
#6483=ORIENTED_EDGE('',*,*,#5099,.F.) ;
#6484=ORIENTED_EDGE('',*,*,#5100,.F.) ;
#6485=ORIENTED_EDGE('',*,*,#5101,.F.) ;
#6486=ORIENTED_EDGE('',*,*,#5102,.T.) ;
#6487=ORIENTED_EDGE('',*,*,#5103,.F.) ;
#6488=ORIENTED_EDGE('',*,*,#5104,.F.) ;
#6489=ORIENTED_EDGE('',*,*,#5102,.F.) ;
#6490=ORIENTED_EDGE('',*,*,#5105,.F.) ;
#6491=ORIENTED_EDGE('',*,*,#5106,.T.) ;
#6492=ORIENTED_EDGE('',*,*,#5107,.T.) ;
#6493=ORIENTED_EDGE('',*,*,#5106,.F.) ;
#6494=ORIENTED_EDGE('',*,*,#5103,.T.) ;
#6495=ORIENTED_EDGE('',*,*,#5104,.T.) ;
#6496=ORIENTED_EDGE('',*,*,#5107,.F.) ;
#6497=ORIENTED_EDGE('',*,*,#5108,.F.) ;
#6498=ORIENTED_EDGE('',*,*,#5109,.T.) ;
#6499=ORIENTED_EDGE('',*,*,#5110,.F.) ;
#6500=ORIENTED_EDGE('',*,*,#5109,.F.) ;
#6501=ORIENTED_EDGE('',*,*,#5111,.F.) ;
#6502=ORIENTED_EDGE('',*,*,#5112,.T.) ;
#6503=ORIENTED_EDGE('',*,*,#5113,.F.) ;
#6504=ORIENTED_EDGE('',*,*,#5112,.F.) ;
#6505=ORIENTED_EDGE('',*,*,#5114,.F.) ;
#6506=ORIENTED_EDGE('',*,*,#5115,.F.) ;
#6507=ORIENTED_EDGE('',*,*,#5116,.F.) ;
#6508=ORIENTED_EDGE('',*,*,#5117,.F.) ;
#6509=ORIENTED_EDGE('',*,*,#5118,.F.) ;
#6510=ORIENTED_EDGE('',*,*,#5119,.F.) ;
#6511=ORIENTED_EDGE('',*,*,#5120,.F.) ;
#6512=ORIENTED_EDGE('',*,*,#5121,.F.) ;
#6513=ORIENTED_EDGE('',*,*,#5120,.T.) ;
#6514=ORIENTED_EDGE('',*,*,#5122,.F.) ;
#6515=ORIENTED_EDGE('',*,*,#5123,.F.) ;
#6516=ORIENTED_EDGE('',*,*,#5124,.T.) ;
#6517=ORIENTED_EDGE('',*,*,#5119,.T.) ;
#6518=ORIENTED_EDGE('',*,*,#5125,.T.) ;
#6519=ORIENTED_EDGE('',*,*,#5126,.T.) ;
#6520=ORIENTED_EDGE('',*,*,#5127,.F.) ;
#6521=ORIENTED_EDGE('',*,*,#5128,.T.) ;
#6522=ORIENTED_EDGE('',*,*,#5122,.T.) ;
#6523=ORIENTED_EDGE('',*,*,#5113,.T.) ;
#6524=ORIENTED_EDGE('',*,*,#5116,.T.) ;
#6525=ORIENTED_EDGE('',*,*,#5129,.F.) ;
#6526=ORIENTED_EDGE('',*,*,#5130,.F.) ;
#6527=ORIENTED_EDGE('',*,*,#5131,.T.) ;
#6528=ORIENTED_EDGE('',*,*,#5115,.T.) ;
#6529=ORIENTED_EDGE('',*,*,#5132,.T.) ;
#6530=ORIENTED_EDGE('',*,*,#5133,.T.) ;
#6531=ORIENTED_EDGE('',*,*,#5134,.F.) ;
#6532=ORIENTED_EDGE('',*,*,#5135,.T.) ;
#6533=ORIENTED_EDGE('',*,*,#5129,.T.) ;
#6534=ORIENTED_EDGE('',*,*,#5110,.T.) ;
#6535=ORIENTED_EDGE('',*,*,#5136,.T.) ;
#6536=ORIENTED_EDGE('',*,*,#5137,.T.) ;
#6537=ORIENTED_EDGE('',*,*,#5138,.T.) ;
#6538=ORIENTED_EDGE('',*,*,#5139,.T.) ;
#6539=ORIENTED_EDGE('',*,*,#5139,.F.) ;
#6540=ORIENTED_EDGE('',*,*,#5140,.F.) ;
#6541=ORIENTED_EDGE('',*,*,#5141,.T.) ;
#6542=ORIENTED_EDGE('',*,*,#5142,.T.) ;
#6543=ORIENTED_EDGE('',*,*,#5143,.T.) ;
#6544=ORIENTED_EDGE('',*,*,#5144,.T.) ;
#6545=ORIENTED_EDGE('',*,*,#5090,.T.) ;
#6546=ORIENTED_EDGE('',*,*,#5138,.F.) ;
#6547=ORIENTED_EDGE('',*,*,#5145,.F.) ;
#6548=ORIENTED_EDGE('',*,*,#5146,.T.) ;
#6549=ORIENTED_EDGE('',*,*,#5147,.T.) ;
#6550=ORIENTED_EDGE('',*,*,#5148,.T.) ;
#6551=ORIENTED_EDGE('',*,*,#5149,.F.) ;
#6552=ORIENTED_EDGE('',*,*,#5150,.T.) ;
#6553=ORIENTED_EDGE('',*,*,#5151,.T.) ;
#6554=ORIENTED_EDGE('',*,*,#5152,.T.) ;
#6555=ORIENTED_EDGE('',*,*,#5153,.F.) ;
#6556=ORIENTED_EDGE('',*,*,#5154,.F.) ;
#6557=ORIENTED_EDGE('',*,*,#5155,.F.) ;
#6558=ORIENTED_EDGE('',*,*,#5156,.F.) ;
#6559=ORIENTED_EDGE('',*,*,#5157,.F.) ;
#6560=ORIENTED_EDGE('',*,*,#5053,.T.) ;
#6561=ORIENTED_EDGE('',*,*,#5158,.T.) ;
#6562=ORIENTED_EDGE('',*,*,#5159,.T.) ;
#6563=ORIENTED_EDGE('',*,*,#5160,.F.) ;
#6564=ORIENTED_EDGE('',*,*,#5043,.T.) ;
#6565=ORIENTED_EDGE('',*,*,#5161,.T.) ;
#6566=ORIENTED_EDGE('',*,*,#5162,.F.) ;
#6567=ORIENTED_EDGE('',*,*,#5140,.T.) ;
#6568=ORIENTED_EDGE('',*,*,#5154,.T.) ;
#6569=ORIENTED_EDGE('',*,*,#5163,.T.) ;
#6570=ORIENTED_EDGE('',*,*,#5164,.T.) ;
#6571=ORIENTED_EDGE('',*,*,#5165,.T.) ;
#6572=ORIENTED_EDGE('',*,*,#5165,.F.) ;
#6573=ORIENTED_EDGE('',*,*,#5166,.F.) ;
#6574=ORIENTED_EDGE('',*,*,#5167,.T.) ;
#6575=ORIENTED_EDGE('',*,*,#5168,.T.) ;
#6576=ORIENTED_EDGE('',*,*,#5169,.T.) ;
#6577=ORIENTED_EDGE('',*,*,#5155,.T.) ;
#6578=ORIENTED_EDGE('',*,*,#5083,.T.) ;
#6579=ORIENTED_EDGE('',*,*,#5170,.F.) ;
#6580=ORIENTED_EDGE('',*,*,#5171,.T.) ;
#6581=ORIENTED_EDGE('',*,*,#5172,.T.) ;
#6582=ORIENTED_EDGE('',*,*,#5173,.F.) ;
#6583=ORIENTED_EDGE('',*,*,#5174,.F.) ;
#6584=ORIENTED_EDGE('',*,*,#5152,.F.) ;
#6585=ORIENTED_EDGE('',*,*,#5175,.T.) ;
#6586=ORIENTED_EDGE('',*,*,#5150,.F.) ;
#6587=ORIENTED_EDGE('',*,*,#5176,.F.) ;
#6588=ORIENTED_EDGE('',*,*,#5177,.F.) ;
#6589=ORIENTED_EDGE('',*,*,#5178,.T.) ;
#6590=ORIENTED_EDGE('',*,*,#5171,.F.) ;
#6591=ORIENTED_EDGE('',*,*,#5092,.T.) ;
#6592=ORIENTED_EDGE('',*,*,#5093,.T.) ;
#6593=ORIENTED_EDGE('',*,*,#5151,.F.) ;
#6594=ORIENTED_EDGE('',*,*,#5175,.F.) ;
#6595=ORIENTED_EDGE('',*,*,#5179,.F.) ;
#6596=ORIENTED_EDGE('',*,*,#5172,.F.) ;
#6597=ORIENTED_EDGE('',*,*,#5178,.F.) ;
#6598=ORIENTED_EDGE('',*,*,#5170,.T.) ;
#6599=ORIENTED_EDGE('',*,*,#5097,.T.) ;
#6600=ORIENTED_EDGE('',*,*,#5173,.T.) ;
#6601=ORIENTED_EDGE('',*,*,#5179,.T.) ;
#6602=ORIENTED_EDGE('',*,*,#5177,.T.) ;
#6603=ORIENTED_EDGE('',*,*,#5180,.F.) ;
#6604=ORIENTED_EDGE('',*,*,#5181,.T.) ;
#6605=ORIENTED_EDGE('',*,*,#5182,.T.) ;
#6606=ORIENTED_EDGE('',*,*,#5183,.T.) ;
#6607=ORIENTED_EDGE('',*,*,#5184,.F.) ;
#6608=ORIENTED_EDGE('',*,*,#5185,.F.) ;
#6609=ORIENTED_EDGE('',*,*,#5186,.T.) ;
#6610=ORIENTED_EDGE('',*,*,#5187,.T.) ;
#6611=ORIENTED_EDGE('',*,*,#5188,.T.) ;
#6612=ORIENTED_EDGE('',*,*,#5189,.F.) ;
#6613=ORIENTED_EDGE('',*,*,#5190,.F.) ;
#6614=ORIENTED_EDGE('',*,*,#5191,.T.) ;
#6615=ORIENTED_EDGE('',*,*,#5192,.T.) ;
#6616=ORIENTED_EDGE('',*,*,#5193,.T.) ;
#6617=ORIENTED_EDGE('',*,*,#5134,.T.) ;
#6618=ORIENTED_EDGE('',*,*,#5194,.T.) ;
#6619=ORIENTED_EDGE('',*,*,#5195,.T.) ;
#6620=ORIENTED_EDGE('',*,*,#5196,.T.) ;
#6621=ORIENTED_EDGE('',*,*,#5127,.T.) ;
#6622=ORIENTED_EDGE('',*,*,#5176,.T.) ;
#6623=ORIENTED_EDGE('',*,*,#5149,.T.) ;
#6624=ORIENTED_EDGE('',*,*,#5197,.T.) ;
#6625=ORIENTED_EDGE('',*,*,#5180,.T.) ;
#6626=ORIENTED_EDGE('',*,*,#5198,.T.) ;
#6627=ORIENTED_EDGE('',*,*,#5123,.T.) ;
#6628=ORIENTED_EDGE('',*,*,#5128,.F.) ;
#6629=ORIENTED_EDGE('',*,*,#5196,.F.) ;
#6630=ORIENTED_EDGE('',*,*,#5199,.T.) ;
#6631=ORIENTED_EDGE('',*,*,#5194,.F.) ;
#6632=ORIENTED_EDGE('',*,*,#5126,.F.) ;
#6633=ORIENTED_EDGE('',*,*,#5200,.F.) ;
#6634=ORIENTED_EDGE('',*,*,#5118,.T.) ;
#6635=ORIENTED_EDGE('',*,*,#5201,.T.) ;
#6636=ORIENTED_EDGE('',*,*,#5200,.T.) ;
#6637=ORIENTED_EDGE('',*,*,#5125,.F.) ;
#6638=ORIENTED_EDGE('',*,*,#5121,.T.) ;
#6639=ORIENTED_EDGE('',*,*,#5124,.F.) ;
#6640=ORIENTED_EDGE('',*,*,#5198,.F.) ;
#6641=ORIENTED_EDGE('',*,*,#5195,.F.) ;
#6642=ORIENTED_EDGE('',*,*,#5199,.F.) ;
#6643=ORIENTED_EDGE('',*,*,#5201,.F.) ;
#6644=ORIENTED_EDGE('',*,*,#5111,.T.) ;
#6645=ORIENTED_EDGE('',*,*,#5202,.F.) ;
#6646=ORIENTED_EDGE('',*,*,#5203,.F.) ;
#6647=ORIENTED_EDGE('',*,*,#5204,.T.) ;
#6648=ORIENTED_EDGE('',*,*,#5205,.T.) ;
#6649=ORIENTED_EDGE('',*,*,#5206,.F.) ;
#6650=ORIENTED_EDGE('',*,*,#5205,.F.) ;
#6651=ORIENTED_EDGE('',*,*,#5207,.F.) ;
#6652=ORIENTED_EDGE('',*,*,#5208,.T.) ;
#6653=ORIENTED_EDGE('',*,*,#5209,.T.) ;
#6654=ORIENTED_EDGE('',*,*,#5207,.T.) ;
#6655=ORIENTED_EDGE('',*,*,#5204,.F.) ;
#6656=ORIENTED_EDGE('',*,*,#5210,.F.) ;
#6657=ORIENTED_EDGE('',*,*,#5211,.F.) ;
#6658=ORIENTED_EDGE('',*,*,#5212,.T.) ;
#6659=ORIENTED_EDGE('',*,*,#5213,.T.) ;
#6660=ORIENTED_EDGE('',*,*,#5181,.F.) ;
#6661=ORIENTED_EDGE('',*,*,#5197,.F.) ;
#6662=ORIENTED_EDGE('',*,*,#5148,.F.) ;
#6663=ORIENTED_EDGE('',*,*,#5214,.T.) ;
#6664=ORIENTED_EDGE('',*,*,#5146,.F.) ;
#6665=ORIENTED_EDGE('',*,*,#5215,.F.) ;
#6666=ORIENTED_EDGE('',*,*,#5183,.F.) ;
#6667=ORIENTED_EDGE('',*,*,#5216,.T.) ;
#6668=ORIENTED_EDGE('',*,*,#5212,.F.) ;
#6669=ORIENTED_EDGE('',*,*,#5100,.T.) ;
#6670=ORIENTED_EDGE('',*,*,#5101,.T.) ;
#6671=ORIENTED_EDGE('',*,*,#5147,.F.) ;
#6672=ORIENTED_EDGE('',*,*,#5214,.F.) ;
#6673=ORIENTED_EDGE('',*,*,#5182,.F.) ;
#6674=ORIENTED_EDGE('',*,*,#5213,.F.) ;
#6675=ORIENTED_EDGE('',*,*,#5216,.F.) ;
#6676=ORIENTED_EDGE('',*,*,#5211,.T.) ;
#6677=ORIENTED_EDGE('',*,*,#5105,.T.) ;
#6678=ORIENTED_EDGE('',*,*,#5217,.T.) ;
#6679=ORIENTED_EDGE('',*,*,#5130,.T.) ;
#6680=ORIENTED_EDGE('',*,*,#5135,.F.) ;
#6681=ORIENTED_EDGE('',*,*,#5193,.F.) ;
#6682=ORIENTED_EDGE('',*,*,#5218,.T.) ;
#6683=ORIENTED_EDGE('',*,*,#5191,.F.) ;
#6684=ORIENTED_EDGE('',*,*,#5133,.F.) ;
#6685=ORIENTED_EDGE('',*,*,#5219,.F.) ;
#6686=ORIENTED_EDGE('',*,*,#5114,.T.) ;
#6687=ORIENTED_EDGE('',*,*,#5220,.T.) ;
#6688=ORIENTED_EDGE('',*,*,#5219,.T.) ;
#6689=ORIENTED_EDGE('',*,*,#5132,.F.) ;
#6690=ORIENTED_EDGE('',*,*,#5117,.T.) ;
#6691=ORIENTED_EDGE('',*,*,#5131,.F.) ;
#6692=ORIENTED_EDGE('',*,*,#5217,.F.) ;
#6693=ORIENTED_EDGE('',*,*,#5192,.F.) ;
#6694=ORIENTED_EDGE('',*,*,#5218,.F.) ;
#6695=ORIENTED_EDGE('',*,*,#5220,.F.) ;
#6696=ORIENTED_EDGE('',*,*,#5108,.T.) ;
#6697=ORIENTED_EDGE('',*,*,#5221,.F.) ;
#6698=ORIENTED_EDGE('',*,*,#5222,.T.) ;
#6699=ORIENTED_EDGE('',*,*,#5223,.T.) ;
#6700=ORIENTED_EDGE('',*,*,#5224,.F.) ;
#6701=ORIENTED_EDGE('',*,*,#5225,.F.) ;
#6702=ORIENTED_EDGE('',*,*,#5226,.T.) ;
#6703=ORIENTED_EDGE('',*,*,#5227,.T.) ;
#6704=ORIENTED_EDGE('',*,*,#5222,.F.) ;
#6705=ORIENTED_EDGE('',*,*,#5228,.T.) ;
#6706=ORIENTED_EDGE('',*,*,#5229,.F.) ;
#6707=ORIENTED_EDGE('',*,*,#5223,.F.) ;
#6708=ORIENTED_EDGE('',*,*,#5227,.F.) ;
#6709=ORIENTED_EDGE('',*,*,#5167,.F.) ;
#6710=ORIENTED_EDGE('',*,*,#5230,.T.) ;
#6711=ORIENTED_EDGE('',*,*,#5231,.T.) ;
#6712=ORIENTED_EDGE('',*,*,#5232,.T.) ;
#6713=ORIENTED_EDGE('',*,*,#5022,.T.) ;
#6714=ORIENTED_EDGE('',*,*,#5233,.T.) ;
#6715=ORIENTED_EDGE('',*,*,#5234,.F.) ;
#6716=ORIENTED_EDGE('',*,*,#5235,.F.) ;
#6717=ORIENTED_EDGE('',*,*,#5023,.T.) ;
#6718=ORIENTED_EDGE('',*,*,#5235,.T.) ;
#6719=ORIENTED_EDGE('',*,*,#5236,.F.) ;
#6720=ORIENTED_EDGE('',*,*,#5232,.F.) ;
#6721=ORIENTED_EDGE('',*,*,#5237,.F.) ;
#6722=ORIENTED_EDGE('',*,*,#5024,.T.) ;
#6723=ORIENTED_EDGE('',*,*,#5237,.T.) ;
#6724=ORIENTED_EDGE('',*,*,#5231,.F.) ;
#6725=ORIENTED_EDGE('',*,*,#5238,.F.) ;
#6726=ORIENTED_EDGE('',*,*,#5143,.F.) ;
#6727=ORIENTED_EDGE('',*,*,#5239,.T.) ;
#6728=ORIENTED_EDGE('',*,*,#5240,.T.) ;
#6729=ORIENTED_EDGE('',*,*,#5241,.T.) ;
#6730=ORIENTED_EDGE('',*,*,#5032,.T.) ;
#6731=ORIENTED_EDGE('',*,*,#5242,.T.) ;
#6732=ORIENTED_EDGE('',*,*,#5240,.F.) ;
#6733=ORIENTED_EDGE('',*,*,#5243,.F.) ;
#6734=ORIENTED_EDGE('',*,*,#5033,.T.) ;
#6735=ORIENTED_EDGE('',*,*,#5243,.T.) ;
#6736=ORIENTED_EDGE('',*,*,#5239,.F.) ;
#6737=ORIENTED_EDGE('',*,*,#5244,.F.) ;
#6738=ORIENTED_EDGE('',*,*,#5245,.F.) ;
#6739=ORIENTED_EDGE('',*,*,#5034,.T.) ;
#6740=ORIENTED_EDGE('',*,*,#5245,.T.) ;
#6741=ORIENTED_EDGE('',*,*,#5246,.F.) ;
#6742=ORIENTED_EDGE('',*,*,#5247,.F.) ;
#6743=ORIENTED_EDGE('',*,*,#5234,.T.) ;
#6744=ORIENTED_EDGE('',*,*,#5248,.F.) ;
#6745=ORIENTED_EDGE('',*,*,#5246,.T.) ;
#6746=ORIENTED_EDGE('',*,*,#5244,.T.) ;
#6747=ORIENTED_EDGE('',*,*,#5142,.F.) ;
#6748=ORIENTED_EDGE('',*,*,#5249,.T.) ;
#6749=ORIENTED_EDGE('',*,*,#5250,.F.) ;
#6750=ORIENTED_EDGE('',*,*,#5228,.F.) ;
#6751=ORIENTED_EDGE('',*,*,#5226,.F.) ;
#6752=ORIENTED_EDGE('',*,*,#5251,.F.) ;
#6753=ORIENTED_EDGE('',*,*,#5208,.F.) ;
#6754=ORIENTED_EDGE('',*,*,#5209,.F.) ;
#6755=ORIENTED_EDGE('',*,*,#5252,.F.) ;
#6756=ORIENTED_EDGE('',*,*,#5253,.T.) ;
#6757=ORIENTED_EDGE('',*,*,#5168,.F.) ;
#6758=ORIENTED_EDGE('',*,*,#5236,.T.) ;
#6759=ORIENTED_EDGE('',*,*,#5206,.T.) ;
#6760=ORIENTED_EDGE('',*,*,#5251,.T.) ;
#6761=ORIENTED_EDGE('',*,*,#5225,.T.) ;
#6762=ORIENTED_EDGE('',*,*,#5221,.T.) ;
#6763=ORIENTED_EDGE('',*,*,#5254,.F.) ;
#6764=ORIENTED_EDGE('',*,*,#5255,.F.) ;
#6765=ORIENTED_EDGE('',*,*,#5256,.F.) ;
#6766=ORIENTED_EDGE('',*,*,#5202,.T.) ;
#6767=ORIENTED_EDGE('',*,*,#5229,.T.) ;
#6768=ORIENTED_EDGE('',*,*,#5250,.T.) ;
#6769=ORIENTED_EDGE('',*,*,#5257,.T.) ;
#6770=ORIENTED_EDGE('',*,*,#5185,.T.) ;
#6771=ORIENTED_EDGE('',*,*,#5258,.F.) ;
#6772=ORIENTED_EDGE('',*,*,#5254,.T.) ;
#6773=ORIENTED_EDGE('',*,*,#5224,.T.) ;
#6774=ORIENTED_EDGE('',*,*,#5088,.T.) ;
#6775=ORIENTED_EDGE('',*,*,#5169,.F.) ;
#6776=ORIENTED_EDGE('',*,*,#5259,.T.) ;
#6777=ORIENTED_EDGE('',*,*,#5260,.T.) ;
#6778=ORIENTED_EDGE('',*,*,#5156,.T.) ;
#6779=ORIENTED_EDGE('',*,*,#5052,.T.) ;
#6780=ORIENTED_EDGE('',*,*,#5261,.T.) ;
#6781=ORIENTED_EDGE('',*,*,#5262,.F.) ;
#6782=ORIENTED_EDGE('',*,*,#5263,.F.) ;
#6783=ORIENTED_EDGE('',*,*,#5158,.F.) ;
#6784=ORIENTED_EDGE('',*,*,#5054,.T.) ;
#6785=ORIENTED_EDGE('',*,*,#5157,.T.) ;
#6786=ORIENTED_EDGE('',*,*,#5260,.F.) ;
#6787=ORIENTED_EDGE('',*,*,#5264,.F.) ;
#6788=ORIENTED_EDGE('',*,*,#5051,.T.) ;
#6789=ORIENTED_EDGE('',*,*,#5264,.T.) ;
#6790=ORIENTED_EDGE('',*,*,#5259,.F.) ;
#6791=ORIENTED_EDGE('',*,*,#5253,.F.) ;
#6792=ORIENTED_EDGE('',*,*,#5265,.F.) ;
#6793=ORIENTED_EDGE('',*,*,#5261,.F.) ;
#6794=ORIENTED_EDGE('',*,*,#5188,.F.) ;
#6795=ORIENTED_EDGE('',*,*,#5262,.T.) ;
#6796=ORIENTED_EDGE('',*,*,#5265,.T.) ;
#6797=ORIENTED_EDGE('',*,*,#5266,.F.) ;
#6798=ORIENTED_EDGE('',*,*,#5263,.T.) ;
#6799=ORIENTED_EDGE('',*,*,#5187,.F.) ;
#6800=ORIENTED_EDGE('',*,*,#5267,.T.) ;
#6801=ORIENTED_EDGE('',*,*,#5159,.F.) ;
#6802=ORIENTED_EDGE('',*,*,#5141,.F.) ;
#6803=ORIENTED_EDGE('',*,*,#5162,.T.) ;
#6804=ORIENTED_EDGE('',*,*,#5268,.T.) ;
#6805=ORIENTED_EDGE('',*,*,#5269,.T.) ;
#6806=ORIENTED_EDGE('',*,*,#5186,.F.) ;
#6807=ORIENTED_EDGE('',*,*,#5257,.F.) ;
#6808=ORIENTED_EDGE('',*,*,#5270,.T.) ;
#6809=ORIENTED_EDGE('',*,*,#5271,.T.) ;
#6810=ORIENTED_EDGE('',*,*,#5042,.T.) ;
#6811=ORIENTED_EDGE('',*,*,#5272,.T.) ;
#6812=ORIENTED_EDGE('',*,*,#5268,.F.) ;
#6813=ORIENTED_EDGE('',*,*,#5161,.F.) ;
#6814=ORIENTED_EDGE('',*,*,#5044,.T.) ;
#6815=ORIENTED_EDGE('',*,*,#5160,.T.) ;
#6816=ORIENTED_EDGE('',*,*,#5267,.F.) ;
#6817=ORIENTED_EDGE('',*,*,#5271,.F.) ;
#6818=ORIENTED_EDGE('',*,*,#5273,.F.) ;
#6819=ORIENTED_EDGE('',*,*,#5041,.T.) ;
#6820=ORIENTED_EDGE('',*,*,#5273,.T.) ;
#6821=ORIENTED_EDGE('',*,*,#5270,.F.) ;
#6822=ORIENTED_EDGE('',*,*,#5249,.F.) ;
#6823=ORIENTED_EDGE('',*,*,#5269,.F.) ;
#6824=ORIENTED_EDGE('',*,*,#5272,.F.) ;
#6825=ORIENTED_EDGE('',*,*,#5203,.T.) ;
#6826=ORIENTED_EDGE('',*,*,#5256,.T.) ;
#6827=ORIENTED_EDGE('',*,*,#5274,.F.) ;
#6828=ORIENTED_EDGE('',*,*,#5189,.T.) ;
#6829=ORIENTED_EDGE('',*,*,#5266,.T.) ;
#6830=ORIENTED_EDGE('',*,*,#5252,.T.) ;
#6831=ORIENTED_EDGE('',*,*,#5210,.T.) ;
#6832=ORIENTED_EDGE('',*,*,#5085,.T.) ;
#6833=ORIENTED_EDGE('',*,*,#5136,.F.) ;
#6834=ORIENTED_EDGE('',*,*,#5144,.F.) ;
#6835=ORIENTED_EDGE('',*,*,#5241,.F.) ;
#6836=ORIENTED_EDGE('',*,*,#5242,.F.) ;
#6837=ORIENTED_EDGE('',*,*,#5031,.T.) ;
#6838=ORIENTED_EDGE('',*,*,#5247,.T.) ;
#6839=ORIENTED_EDGE('',*,*,#5248,.T.) ;
#6840=ORIENTED_EDGE('',*,*,#5233,.F.) ;
#6841=ORIENTED_EDGE('',*,*,#5021,.T.) ;
#6842=ORIENTED_EDGE('',*,*,#5238,.T.) ;
#6843=ORIENTED_EDGE('',*,*,#5230,.F.) ;
#6844=ORIENTED_EDGE('',*,*,#5166,.T.) ;
#6845=ORIENTED_EDGE('',*,*,#5164,.F.) ;
#6846=ORIENTED_EDGE('',*,*,#5275,.F.) ;
#6847=ORIENTED_EDGE('',*,*,#5137,.F.) ;
#6848=ORIENTED_EDGE('',*,*,#5275,.T.) ;
#6849=ORIENTED_EDGE('',*,*,#5163,.F.) ;
#6850=ORIENTED_EDGE('',*,*,#5153,.T.) ;
#6851=ORIENTED_EDGE('',*,*,#5174,.T.) ;
#6852=ORIENTED_EDGE('',*,*,#5190,.T.) ;
#6853=ORIENTED_EDGE('',*,*,#5274,.T.) ;
#6854=ORIENTED_EDGE('',*,*,#5255,.T.) ;
#6855=ORIENTED_EDGE('',*,*,#5258,.T.) ;
#6856=ORIENTED_EDGE('',*,*,#5184,.T.) ;
#6857=ORIENTED_EDGE('',*,*,#5215,.T.) ;
#6858=ORIENTED_EDGE('',*,*,#5145,.T.) ;
#8993=CONICAL_SURFACE('',#9749,1.12500000000001,0.785398163397463) ;
#8994=CONICAL_SURFACE('',#9756,1.12500000000001,0.785398163397463) ;
#8995=CONICAL_SURFACE('',#9763,1.12500000000001,0.785398163397463) ;
#8996=CONICAL_SURFACE('',#9770,1.12500000000001,0.785398163397463) ;
#8997=CONICAL_SURFACE('',#9777,1.125,0.785398163397434) ;
#8998=CONICAL_SURFACE('',#9782,1.125,0.785398163397434) ;
#8999=CONICAL_SURFACE('',#9787,1.125,0.785398163397434) ;
#9000=CONICAL_SURFACE('',#9791,1.125,0.785398163397434) ;
#9001=CONICAL_SURFACE('',#9795,1.04999999999999,1.02974425867665) ;
#9002=CONICAL_SURFACE('',#9796,1.05,1.02974425867665) ;
#9003=CONICAL_SURFACE('',#9797,1.04999999999999,1.02974425867665) ;
#9004=CONICAL_SURFACE('',#9798,1.05,1.02974425867665) ;
#9005=CONICAL_SURFACE('',#9799,1.05,1.02974425867665) ;
#9006=CONICAL_SURFACE('',#9803,1.05,1.02974425867666) ;
#9007=CONICAL_SURFACE('',#9804,1.05,1.02974425867665) ;
#9008=CONICAL_SURFACE('',#9808,1.05,1.02974425867666) ;
#9023=ADVANCED_FACE('',(#1087),#8993,.F.) ;
#9024=ADVANCED_FACE('',(#1088,#651,#652),#759,.F.) ;
#9025=ADVANCED_FACE('',(#1089),#500,.F.) ;
#9026=ADVANCED_FACE('',(#1090),#8994,.F.) ;
#9027=ADVANCED_FACE('',(#1091,#653,#654),#760,.F.) ;
#9028=ADVANCED_FACE('',(#1092),#501,.F.) ;
#9029=ADVANCED_FACE('',(#1093),#8995,.F.) ;
#9030=ADVANCED_FACE('',(#1094,#655,#656),#761,.F.) ;
#9031=ADVANCED_FACE('',(#1095),#502,.F.) ;
#9032=ADVANCED_FACE('',(#1096),#8996,.F.) ;
#9033=ADVANCED_FACE('',(#1097,#657,#658),#762,.F.) ;
#9034=ADVANCED_FACE('',(#1098),#503,.F.) ;
#9035=ADVANCED_FACE('',(#1099),#8997,.F.) ;
#9036=ADVANCED_FACE('',(#1100),#504,.F.) ;
#9037=ADVANCED_FACE('',(#1101),#8998,.F.) ;
#9038=ADVANCED_FACE('',(#1102),#505,.F.) ;
#9039=ADVANCED_FACE('',(#1103),#8999,.F.) ;
#9040=ADVANCED_FACE('',(#1104),#506,.F.) ;
#9041=ADVANCED_FACE('',(#1105),#9000,.F.) ;
#9042=ADVANCED_FACE('',(#1106),#507,.F.) ;
#9043=ADVANCED_FACE('',(#1107),#9001,.F.) ;
#9044=ADVANCED_FACE('',(#1108),#9002,.F.) ;
#9045=ADVANCED_FACE('',(#1109),#9003,.F.) ;
#9046=ADVANCED_FACE('',(#1110),#9004,.F.) ;
#9047=ADVANCED_FACE('',(#1111),#9005,.F.) ;
#9048=ADVANCED_FACE('',(#1112,#659),#508,.F.) ;
#9049=ADVANCED_FACE('',(#1113),#9006,.F.) ;
#9050=ADVANCED_FACE('',(#1114),#9007,.F.) ;
#9051=ADVANCED_FACE('',(#1115,#660),#509,.F.) ;
#9052=ADVANCED_FACE('',(#1116),#9008,.F.) ;
#9053=ADVANCED_FACE('',(#1117),#510,.F.) ;
#9054=ADVANCED_FACE('',(#1118,#661),#511,.F.) ;
#9055=ADVANCED_FACE('',(#1119),#763,.T.) ;
#9056=ADVANCED_FACE('',(#1120),#512,.F.) ;
#9057=ADVANCED_FACE('',(#1121,#662),#513,.F.) ;
#9058=ADVANCED_FACE('',(#1122),#764,.T.) ;
#9059=ADVANCED_FACE('',(#1123),#514,.F.) ;
#9060=ADVANCED_FACE('',(#1124),#515,.F.) ;
#9061=ADVANCED_FACE('',(#1125),#516,.F.) ;
#9062=ADVANCED_FACE('',(#1126),#517,.F.) ;
#9063=ADVANCED_FACE('',(#1127),#765,.T.) ;
#9064=ADVANCED_FACE('',(#1128,#663),#766,.T.) ;
#9065=ADVANCED_FACE('',(#1129),#767,.T.) ;
#9066=ADVANCED_FACE('',(#1130,#664),#768,.T.) ;
#9067=ADVANCED_FACE('',(#1131),#769,.T.) ;
#9068=ADVANCED_FACE('',(#1132,#665),#770,.T.) ;
#9069=ADVANCED_FACE('',(#1133),#771,.T.) ;
#9070=ADVANCED_FACE('',(#1134),#772,.T.) ;
#9071=ADVANCED_FACE('',(#1135,#666),#773,.T.) ;
#9072=ADVANCED_FACE('',(#1136,#667),#518,.T.) ;
#9073=ADVANCED_FACE('',(#1137),#774,.T.) ;
#9074=ADVANCED_FACE('',(#1138),#775,.T.) ;
#9075=ADVANCED_FACE('',(#1139,#668),#776,.T.) ;
#9076=ADVANCED_FACE('',(#1140,#669,#670),#777,.T.) ;
#9077=ADVANCED_FACE('',(#1141),#778,.T.) ;
#9078=ADVANCED_FACE('',(#1142),#779,.T.) ;
#9079=ADVANCED_FACE('',(#1143),#780,.T.) ;
#9080=ADVANCED_FACE('',(#1144),#519,.T.) ;
#9081=ADVANCED_FACE('',(#1145,#671),#781,.F.) ;
#9082=ADVANCED_FACE('',(#1146),#782,.T.) ;
#9083=ADVANCED_FACE('',(#1147),#783,.T.) ;
#9084=ADVANCED_FACE('',(#1148),#784,.T.) ;
#9085=ADVANCED_FACE('',(#1149,#672),#520,.T.) ;
#9086=ADVANCED_FACE('',(#1150),#785,.T.) ;
#9087=ADVANCED_FACE('',(#1151),#786,.T.) ;
#9088=ADVANCED_FACE('',(#1152,#673),#787,.T.) ;
#9089=ADVANCED_FACE('',(#1153),#788,.T.) ;
#9090=ADVANCED_FACE('',(#1154),#789,.T.) ;
#9091=ADVANCED_FACE('',(#1155),#521,.T.) ;
#9092=ADVANCED_FACE('',(#1156,#674),#790,.F.) ;
#9093=ADVANCED_FACE('',(#1157),#791,.T.) ;
#9094=ADVANCED_FACE('',(#1158),#792,.T.) ;
#9095=ADVANCED_FACE('',(#1159),#793,.T.) ;
#9096=ADVANCED_FACE('',(#1160),#794,.T.) ;
#9097=ADVANCED_FACE('',(#1161),#795,.T.) ;
#9098=ADVANCED_FACE('',(#1162),#796,.T.) ;
#9099=ADVANCED_FACE('',(#1163),#797,.T.) ;
#9100=ADVANCED_FACE('',(#1164),#798,.T.) ;
#9101=ADVANCED_FACE('',(#1165),#799,.T.) ;
#9102=ADVANCED_FACE('',(#1166),#800,.T.) ;
#9103=ADVANCED_FACE('',(#1167),#801,.T.) ;
#9104=ADVANCED_FACE('',(#1168),#802,.F.) ;
#9105=ADVANCED_FACE('',(#1169),#803,.T.) ;
#9106=ADVANCED_FACE('',(#1170,#675),#804,.T.) ;
#9107=ADVANCED_FACE('',(#1171),#805,.T.) ;
#9108=ADVANCED_FACE('',(#1172),#806,.T.) ;
#9109=ADVANCED_FACE('',(#1173),#807,.T.) ;
#9110=ADVANCED_FACE('',(#1174),#808,.T.) ;
#9111=ADVANCED_FACE('',(#1175),#809,.T.) ;
#9112=ADVANCED_FACE('',(#1176),#810,.F.) ;
#9113=ADVANCED_FACE('',(#1177),#811,.T.) ;
#9114=ADVANCED_FACE('',(#1178),#812,.T.) ;
#9115=ADVANCED_FACE('',(#1179),#813,.T.) ;
#9116=ADVANCED_FACE('',(#1180),#814,.T.) ;
#9117=ADVANCED_FACE('',(#1181),#815,.T.) ;
#9118=ADVANCED_FACE('',(#1182,#676),#816,.T.) ;
#9119=ADVANCED_FACE('',(#1183),#817,.T.) ;
#9120=ADVANCED_FACE('',(#1184),#818,.T.) ;
#9542=CLOSED_SHELL('',(#9023,#9024,#9025,#9026,#9027,#9028,#9029,#9030,
#9031,#9032,#9033,#9034,#9035,#9036,#9037,#9038,#9039,#9040,#9041,#9042,
#9043,#9044,#9045,#9046,#9047,#9048,#9049,#9050,#9051,#9052,#9053,#9054,
#9055,#9056,#9057,#9058,#9059,#9060,#9061,#9062,#9063,#9064,#9065,#9066,
#9067,#9068,#9069,#9070,#9071,#9072,#9073,#9074,#9075,#9076,#9077,#9078,
#9079,#9080,#9081,#9082,#9083,#9084,#9085,#9086,#9087,#9088,#9089,#9090,
#9091,#9092,#9093,#9094,#9095,#9096,#9097,#9098,#9099,#9100,#9101,#9102,
#9103,#9104,#9105,#9106,#9107,#9108,#9109,#9110,#9111,#9112,#9113,#9114,
#9115,#9116,#9117,#9118,#9119,#9120)) ;
#9748=AXIS2_PLACEMENT_3D('',#13423,#10717,#10718) ;
#9749=AXIS2_PLACEMENT_3D('',#13424,#10719,#10720) ;
#9750=AXIS2_PLACEMENT_3D('',#13426,#10721,#10722) ;
#9751=AXIS2_PLACEMENT_3D('',#13429,#10724,#10725) ;
#9752=AXIS2_PLACEMENT_3D('',#13430,#10726,#10727) ;
#9753=AXIS2_PLACEMENT_3D('',#13440,#10732,#10733) ;
#9754=AXIS2_PLACEMENT_3D('',#13441,#10734,#10735) ;
#9755=AXIS2_PLACEMENT_3D('',#13444,#10737,#10738) ;
#9756=AXIS2_PLACEMENT_3D('',#13445,#10739,#10740) ;
#9757=AXIS2_PLACEMENT_3D('',#13447,#10741,#10742) ;
#9758=AXIS2_PLACEMENT_3D('',#13450,#10744,#10745) ;
#9759=AXIS2_PLACEMENT_3D('',#13451,#10746,#10747) ;
#9760=AXIS2_PLACEMENT_3D('',#13461,#10752,#10753) ;
#9761=AXIS2_PLACEMENT_3D('',#13462,#10754,#10755) ;
#9762=AXIS2_PLACEMENT_3D('',#13465,#10757,#10758) ;
#9763=AXIS2_PLACEMENT_3D('',#13466,#10759,#10760) ;
#9764=AXIS2_PLACEMENT_3D('',#13468,#10761,#10762) ;
#9765=AXIS2_PLACEMENT_3D('',#13471,#10764,#10765) ;
#9766=AXIS2_PLACEMENT_3D('',#13472,#10766,#10767) ;
#9767=AXIS2_PLACEMENT_3D('',#13482,#10772,#10773) ;
#9768=AXIS2_PLACEMENT_3D('',#13483,#10774,#10775) ;
#9769=AXIS2_PLACEMENT_3D('',#13486,#10777,#10778) ;
#9770=AXIS2_PLACEMENT_3D('',#13487,#10779,#10780) ;
#9771=AXIS2_PLACEMENT_3D('',#13489,#10781,#10782) ;
#9772=AXIS2_PLACEMENT_3D('',#13492,#10784,#10785) ;
#9773=AXIS2_PLACEMENT_3D('',#13493,#10786,#10787) ;
#9774=AXIS2_PLACEMENT_3D('',#13503,#10792,#10793) ;
#9775=AXIS2_PLACEMENT_3D('',#13504,#10794,#10795) ;
#9776=AXIS2_PLACEMENT_3D('',#13507,#10797,#10798) ;
#9777=AXIS2_PLACEMENT_3D('',#13508,#10799,#10800) ;
#9778=AXIS2_PLACEMENT_3D('',#13511,#10802,#10803) ;
#9779=AXIS2_PLACEMENT_3D('',#13512,#10804,#10805) ;
#9780=AXIS2_PLACEMENT_3D('',#13516,#10807,#10808) ;
#9781=AXIS2_PLACEMENT_3D('',#13553,#10809,#10810) ;
#9782=AXIS2_PLACEMENT_3D('',#13554,#10811,#10812) ;
#9783=AXIS2_PLACEMENT_3D('',#13557,#10814,#10815) ;
#9784=AXIS2_PLACEMENT_3D('',#13558,#10816,#10817) ;
#9785=AXIS2_PLACEMENT_3D('',#13562,#10819,#10820) ;
#9786=AXIS2_PLACEMENT_3D('',#13599,#10821,#10822) ;
#9787=AXIS2_PLACEMENT_3D('',#13600,#10823,#10824) ;
#9788=AXIS2_PLACEMENT_3D('',#13603,#10826,#10827) ;
#9789=AXIS2_PLACEMENT_3D('',#13604,#10828,#10829) ;
#9790=AXIS2_PLACEMENT_3D('',#13607,#10831,#10832) ;
#9791=AXIS2_PLACEMENT_3D('',#13608,#10833,#10834) ;
#9792=AXIS2_PLACEMENT_3D('',#13611,#10836,#10837) ;
#9793=AXIS2_PLACEMENT_3D('',#13612,#10838,#10839) ;
#9794=AXIS2_PLACEMENT_3D('',#13615,#10841,#10842) ;
#9795=AXIS2_PLACEMENT_3D('',#13616,#10843,#10844) ;
#9796=AXIS2_PLACEMENT_3D('',#13619,#10846,#10847) ;
#9797=AXIS2_PLACEMENT_3D('',#13622,#10849,#10850) ;
#9798=AXIS2_PLACEMENT_3D('',#13625,#10852,#10853) ;
#9799=AXIS2_PLACEMENT_3D('',#13628,#10855,#10856) ;
#9800=AXIS2_PLACEMENT_3D('',#13636,#10857,#10858) ;
#9801=AXIS2_PLACEMENT_3D('',#13638,#10859,#10860) ;
#9802=AXIS2_PLACEMENT_3D('',#13641,#10862,#10863) ;
#9803=AXIS2_PLACEMENT_3D('',#13642,#10864,#10865) ;
#9804=AXIS2_PLACEMENT_3D('',#13645,#10867,#10868) ;
#9805=AXIS2_PLACEMENT_3D('',#13653,#10869,#10870) ;
#9806=AXIS2_PLACEMENT_3D('',#13655,#10871,#10872) ;
#9807=AXIS2_PLACEMENT_3D('',#13658,#10874,#10875) ;
#9808=AXIS2_PLACEMENT_3D('',#13659,#10876,#10877) ;
#9809=AXIS2_PLACEMENT_3D('',#13662,#10879,#10880) ;
#9810=AXIS2_PLACEMENT_3D('',#13740,#10882,#10883) ;
#9811=AXIS2_PLACEMENT_3D('',#13742,#10884,#10885) ;
#9812=AXIS2_PLACEMENT_3D('',#13745,#10887,#10888) ;
#9813=AXIS2_PLACEMENT_3D('',#13746,#10889,#10890) ;
#9814=AXIS2_PLACEMENT_3D('',#13747,#10891,#10892) ;
#9815=AXIS2_PLACEMENT_3D('',#13825,#10894,#10895) ;
#9816=AXIS2_PLACEMENT_3D('',#13827,#10896,#10897) ;
#9817=AXIS2_PLACEMENT_3D('',#13830,#10899,#10900) ;
#9818=AXIS2_PLACEMENT_3D('',#13831,#10901,#10902) ;
#9819=AXIS2_PLACEMENT_3D('',#13832,#10903,#10904) ;
#9820=AXIS2_PLACEMENT_3D('',#13834,#10905,#10906) ;
#9821=AXIS2_PLACEMENT_3D('',#13837,#10908,#10909) ;
#9822=AXIS2_PLACEMENT_3D('',#13838,#10910,#10911) ;
#9823=AXIS2_PLACEMENT_3D('',#13840,#10912,#10913) ;
#9824=AXIS2_PLACEMENT_3D('',#13843,#10915,#10916) ;
#9825=AXIS2_PLACEMENT_3D('',#13844,#10917,#10918) ;
#9826=AXIS2_PLACEMENT_3D('',#13849,#10920,#10921) ;
#9827=AXIS2_PLACEMENT_3D('',#13852,#10923,#10924) ;
#9828=AXIS2_PLACEMENT_3D('',#13853,#10925,#10926) ;
#9829=AXIS2_PLACEMENT_3D('',#13858,#10928,#10929) ;
#9830=AXIS2_PLACEMENT_3D('',#13861,#10931,#10932) ;
#9831=AXIS2_PLACEMENT_3D('',#13862,#10933,#10934) ;
#9832=AXIS2_PLACEMENT_3D('',#13868,#10938,#10939) ;
#9833=AXIS2_PLACEMENT_3D('',#13870,#10940,#10941) ;
#9834=AXIS2_PLACEMENT_3D('',#13876,#10945,#10946) ;
#9835=AXIS2_PLACEMENT_3D('',#13882,#10950,#10951) ;
#9836=AXIS2_PLACEMENT_3D('',#13884,#10952,#10953) ;
#9837=AXIS2_PLACEMENT_3D('',#13890,#10957,#10958) ;
#9838=AXIS2_PLACEMENT_3D('',#13899,#10963,#10964) ;
#9839=AXIS2_PLACEMENT_3D('',#13909,#10970,#10971) ;
#9840=AXIS2_PLACEMENT_3D('',#13943,#10990,#10991) ;
#9841=AXIS2_PLACEMENT_3D('',#13949,#10995,#10996) ;
#9842=AXIS2_PLACEMENT_3D('',#13957,#11001,#11002) ;
#9843=AXIS2_PLACEMENT_3D('',#13959,#11003,#11004) ;
#9844=AXIS2_PLACEMENT_3D('',#13963,#11006,#11007) ;
#9845=AXIS2_PLACEMENT_3D('',#13966,#11009,#11010) ;
#9846=AXIS2_PLACEMENT_3D('',#13967,#11011,#11012) ;
#9847=AXIS2_PLACEMENT_3D('',#13969,#11013,#11014) ;
#9848=AXIS2_PLACEMENT_3D('',#13972,#11016,#11017) ;
#9849=AXIS2_PLACEMENT_3D('',#13973,#11018,#11019) ;
#9850=AXIS2_PLACEMENT_3D('',#13974,#11020,#11021) ;
#9851=AXIS2_PLACEMENT_3D('',#13976,#11023,#11024) ;
#9852=AXIS2_PLACEMENT_3D('',#13977,#11025,#11026) ;
#9853=AXIS2_PLACEMENT_3D('',#14009,#11044,#11045) ;
#9854=AXIS2_PLACEMENT_3D('',#14010,#11046,#11047) ;
#9855=AXIS2_PLACEMENT_3D('',#14011,#11048,#11049) ;
#9856=AXIS2_PLACEMENT_3D('',#14013,#11051,#11052) ;
#9857=AXIS2_PLACEMENT_3D('',#14017,#11055,#11056) ;
#9858=AXIS2_PLACEMENT_3D('',#14018,#11057,#11058) ;
#9859=AXIS2_PLACEMENT_3D('',#14019,#11059,#11060) ;
#9860=AXIS2_PLACEMENT_3D('',#14020,#11061,#11062) ;
#9861=AXIS2_PLACEMENT_3D('',#14029,#11067,#11068) ;
#9862=AXIS2_PLACEMENT_3D('',#14035,#11072,#11073) ;
#9863=AXIS2_PLACEMENT_3D('',#14039,#11076,#11077) ;
#9864=AXIS2_PLACEMENT_3D('',#14041,#11078,#11079) ;
#9865=AXIS2_PLACEMENT_3D('',#14044,#11081,#11082) ;
#9866=AXIS2_PLACEMENT_3D('',#14045,#11083,#11084) ;
#9867=AXIS2_PLACEMENT_3D('',#14046,#11085,#11086) ;
#9868=AXIS2_PLACEMENT_3D('',#14047,#11087,#11088) ;
#9869=AXIS2_PLACEMENT_3D('',#14048,#11089,#11090) ;
#9870=AXIS2_PLACEMENT_3D('',#14049,#11091,#11092) ;
#9871=AXIS2_PLACEMENT_3D('',#14050,#11093,#11094) ;
#9872=AXIS2_PLACEMENT_3D('',#14051,#11095,#11096) ;
#9873=AXIS2_PLACEMENT_3D('',#14053,#11098,#11099) ;
#9874=AXIS2_PLACEMENT_3D('',#14057,#11102,#11103) ;
#9875=AXIS2_PLACEMENT_3D('',#14058,#11104,#11105) ;
#9876=AXIS2_PLACEMENT_3D('',#14059,#11106,#11107) ;
#9877=AXIS2_PLACEMENT_3D('',#14060,#11108,#11109) ;
#9878=AXIS2_PLACEMENT_3D('',#14069,#11114,#11115) ;
#9879=AXIS2_PLACEMENT_3D('',#14075,#11119,#11120) ;
#9880=AXIS2_PLACEMENT_3D('',#14079,#11123,#11124) ;
#9881=AXIS2_PLACEMENT_3D('',#14085,#11128,#11129) ;
#9882=AXIS2_PLACEMENT_3D('',#14091,#11133,#11134) ;
#9883=AXIS2_PLACEMENT_3D('',#14094,#11137,#11138) ;
#9884=AXIS2_PLACEMENT_3D('',#14096,#11140,#11141) ;
#9885=AXIS2_PLACEMENT_3D('',#14102,#11145,#11146) ;
#9886=AXIS2_PLACEMENT_3D('',#14105,#11149,#11150) ;
#9887=AXIS2_PLACEMENT_3D('',#14109,#11153,#11154) ;
#9888=AXIS2_PLACEMENT_3D('',#14113,#11157,#11158) ;
#9889=AXIS2_PLACEMENT_3D('',#14122,#11165,#11166) ;
#9890=AXIS2_PLACEMENT_3D('',#14128,#11170,#11171) ;
#9891=AXIS2_PLACEMENT_3D('',#14131,#11174,#11175) ;
#9892=AXIS2_PLACEMENT_3D('',#14135,#11178,#11179) ;
#9893=AXIS2_PLACEMENT_3D('',#14140,#11183,#11184) ;
#9894=AXIS2_PLACEMENT_3D('',#14142,#11186,#11187) ;
#9895=AXIS2_PLACEMENT_3D('',#14144,#11189,#11190) ;
#9896=AXIS2_PLACEMENT_3D('',#14146,#11192,#11193) ;
#9897=AXIS2_PLACEMENT_3D('',#14148,#11195,#11196) ;
#9898=AXIS2_PLACEMENT_3D('',#14152,#11199,#11200) ;
#9899=AXIS2_PLACEMENT_3D('',#14156,#11203,#11204) ;
#9900=AXIS2_PLACEMENT_3D('',#14158,#11206,#11207) ;
#9901=AXIS2_PLACEMENT_3D('',#14160,#11209,#11210) ;
#9902=AXIS2_PLACEMENT_3D('',#14161,#11211,#11212) ;
#9903=AXIS2_PLACEMENT_3D('',#14163,#11214,#11215) ;
#9904=AXIS2_PLACEMENT_3D('',#14165,#11217,#11218) ;
#10717=DIRECTION('axis',(0.,0.,1.)) ;
#10718=DIRECTION('refdir',(1.,0.,0.)) ;
#10719=DIRECTION('center_axis',(0.,0.,-1.)) ;
#10720=DIRECTION('ref_axis',(1.,0.,0.)) ;
#10721=DIRECTION('center_axis',(0.,0.,-1.)) ;
#10722=DIRECTION('ref_axis',(1.,0.,0.)) ;
#10723=DIRECTION('',(0.707106781186558,-8.65956056235506E-17,0.707106781186537)) ;
#10724=DIRECTION('center_axis',(0.,0.,1.)) ;
#10725=DIRECTION('ref_axis',(1.,0.,0.)) ;
#10726=DIRECTION('center_axis',(0.,0.,1.)) ;
#10727=DIRECTION('ref_axis',(1.,0.,0.)) ;
#10728=DIRECTION('',(0.,-1.,0.)) ;
#10729=DIRECTION('',(-1.,0.,0.)) ;
#10730=DIRECTION('',(0.,1.,0.)) ;
#10731=DIRECTION('',(1.,0.,0.)) ;
#10732=DIRECTION('center_axis',(0.,0.,-1.)) ;
#10733=DIRECTION('ref_axis',(1.,0.,0.)) ;
#10734=DIRECTION('center_axis',(0.,0.,1.)) ;
#10735=DIRECTION('ref_axis',(1.,0.,0.)) ;
#10736=DIRECTION('',(0.,0.,1.)) ;
#10737=DIRECTION('center_axis',(0.,0.,1.)) ;
#10738=DIRECTION('ref_axis',(1.,0.,0.)) ;
#10739=DIRECTION('center_axis',(0.,0.,-1.)) ;
#10740=DIRECTION('ref_axis',(1.,0.,0.)) ;
#10741=DIRECTION('center_axis',(0.,0.,-1.)) ;
#10742=DIRECTION('ref_axis',(1.,0.,0.)) ;
#10743=DIRECTION('',(0.707106781186558,-8.65956056235506E-17,0.707106781186537)) ;
#10744=DIRECTION('center_axis',(0.,0.,1.)) ;
#10745=DIRECTION('ref_axis',(1.,0.,0.)) ;
#10746=DIRECTION('center_axis',(0.,0.,1.)) ;
#10747=DIRECTION('ref_axis',(1.,0.,0.)) ;
#10748=DIRECTION('',(0.,-1.,0.)) ;
#10749=DIRECTION('',(-1.,0.,0.)) ;
#10750=DIRECTION('',(0.,1.,0.)) ;
#10751=DIRECTION('',(1.,0.,0.)) ;
#10752=DIRECTION('center_axis',(0.,0.,-1.)) ;
#10753=DIRECTION('ref_axis',(1.,0.,0.)) ;
#10754=DIRECTION('center_axis',(0.,0.,1.)) ;
#10755=DIRECTION('ref_axis',(1.,0.,0.)) ;
#10756=DIRECTION('',(0.,0.,1.)) ;
#10757=DIRECTION('center_axis',(0.,0.,1.)) ;
#10758=DIRECTION('ref_axis',(1.,0.,0.)) ;
#10759=DIRECTION('center_axis',(0.,0.,-1.)) ;
#10760=DIRECTION('ref_axis',(1.,0.,0.)) ;
#10761=DIRECTION('center_axis',(0.,0.,-1.)) ;
#10762=DIRECTION('ref_axis',(1.,0.,0.)) ;
#10763=DIRECTION('',(0.707106781186558,-8.65956056235506E-17,0.707106781186537)) ;
#10764=DIRECTION('center_axis',(0.,0.,1.)) ;
#10765=DIRECTION('ref_axis',(1.,0.,0.)) ;
#10766=DIRECTION('center_axis',(0.,0.,1.)) ;
#10767=DIRECTION('ref_axis',(1.,0.,0.)) ;
#10768=DIRECTION('',(0.,-1.,0.)) ;
#10769=DIRECTION('',(-1.,0.,0.)) ;
#10770=DIRECTION('',(0.,1.,0.)) ;
#10771=DIRECTION('',(1.,0.,0.)) ;
#10772=DIRECTION('center_axis',(0.,0.,-1.)) ;
#10773=DIRECTION('ref_axis',(1.,0.,0.)) ;
#10774=DIRECTION('center_axis',(0.,0.,1.)) ;
#10775=DIRECTION('ref_axis',(1.,0.,0.)) ;
#10776=DIRECTION('',(0.,0.,1.)) ;
#10777=DIRECTION('center_axis',(0.,0.,1.)) ;
#10778=DIRECTION('ref_axis',(1.,0.,0.)) ;
#10779=DIRECTION('center_axis',(0.,0.,-1.)) ;
#10780=DIRECTION('ref_axis',(1.,0.,0.)) ;
#10781=DIRECTION('center_axis',(0.,0.,-1.)) ;
#10782=DIRECTION('ref_axis',(1.,0.,0.)) ;
#10783=DIRECTION('',(0.707106781186558,-8.65956056235506E-17,0.707106781186537)) ;
#10784=DIRECTION('center_axis',(0.,0.,1.)) ;
#10785=DIRECTION('ref_axis',(1.,0.,0.)) ;
#10786=DIRECTION('center_axis',(0.,0.,1.)) ;
#10787=DIRECTION('ref_axis',(1.,0.,0.)) ;
#10788=DIRECTION('',(0.,-1.,0.)) ;
#10789=DIRECTION('',(-1.,0.,0.)) ;
#10790=DIRECTION('',(0.,1.,0.)) ;
#10791=DIRECTION('',(1.,0.,0.)) ;
#10792=DIRECTION('center_axis',(0.,0.,-1.)) ;
#10793=DIRECTION('ref_axis',(1.,0.,0.)) ;
#10794=DIRECTION('center_axis',(0.,0.,1.)) ;
#10795=DIRECTION('ref_axis',(1.,0.,0.)) ;
#10796=DIRECTION('',(0.,0.,1.)) ;
#10797=DIRECTION('center_axis',(0.,0.,1.)) ;
#10798=DIRECTION('ref_axis',(1.,0.,0.)) ;
#10799=DIRECTION('center_axis',(0.,0.,-1.)) ;
#10800=DIRECTION('ref_axis',(1.,0.,0.)) ;
#10801=DIRECTION('',(0.707106781186537,-8.6595605623548E-17,0.707106781186558)) ;
#10802=DIRECTION('center_axis',(0.,0.,1.)) ;
#10803=DIRECTION('ref_axis',(1.,0.,0.)) ;
#10804=DIRECTION('center_axis',(0.,0.,1.)) ;
#10805=DIRECTION('ref_axis',(1.,0.,0.)) ;
#10806=DIRECTION('',(0.,0.,1.)) ;
#10807=DIRECTION('center_axis',(0.,0.,1.)) ;
#10808=DIRECTION('ref_axis',(1.,0.,0.)) ;
#10809=DIRECTION('center_axis',(0.,0.,1.)) ;
#10810=DIRECTION('ref_axis',(1.,0.,0.)) ;
#10811=DIRECTION('center_axis',(0.,0.,-1.)) ;
#10812=DIRECTION('ref_axis',(1.,0.,0.)) ;
#10813=DIRECTION('',(0.707106781186537,-8.6595605623548E-17,0.707106781186558)) ;
#10814=DIRECTION('center_axis',(0.,0.,1.)) ;
#10815=DIRECTION('ref_axis',(1.,0.,0.)) ;
#10816=DIRECTION('center_axis',(0.,0.,1.)) ;
#10817=DIRECTION('ref_axis',(1.,0.,0.)) ;
#10818=DIRECTION('',(0.,0.,1.)) ;
#10819=DIRECTION('center_axis',(0.,0.,1.)) ;
#10820=DIRECTION('ref_axis',(1.,0.,0.)) ;
#10821=DIRECTION('center_axis',(0.,0.,1.)) ;
#10822=DIRECTION('ref_axis',(1.,0.,0.)) ;
#10823=DIRECTION('center_axis',(0.,0.,-1.)) ;
#10824=DIRECTION('ref_axis',(1.,0.,0.)) ;
#10825=DIRECTION('',(0.707106781186537,-8.6595605623548E-17,0.707106781186558)) ;
#10826=DIRECTION('center_axis',(0.,0.,1.)) ;
#10827=DIRECTION('ref_axis',(1.,0.,0.)) ;
#10828=DIRECTION('center_axis',(0.,0.,1.)) ;
#10829=DIRECTION('ref_axis',(1.,0.,0.)) ;
#10830=DIRECTION('',(0.,0.,1.)) ;
#10831=DIRECTION('center_axis',(0.,0.,1.)) ;
#10832=DIRECTION('ref_axis',(1.,0.,0.)) ;
#10833=DIRECTION('center_axis',(0.,0.,-1.)) ;
#10834=DIRECTION('ref_axis',(1.,0.,0.)) ;
#10835=DIRECTION('',(0.707106781186537,-8.6595605623548E-17,0.707106781186558)) ;
#10836=DIRECTION('center_axis',(0.,0.,1.)) ;
#10837=DIRECTION('ref_axis',(1.,0.,0.)) ;
#10838=DIRECTION('center_axis',(0.,0.,1.)) ;
#10839=DIRECTION('ref_axis',(1.,0.,0.)) ;
#10840=DIRECTION('',(0.,0.,1.)) ;
#10841=DIRECTION('center_axis',(0.,0.,1.)) ;
#10842=DIRECTION('ref_axis',(1.,0.,0.)) ;
#10843=DIRECTION('center_axis',(0.,0.,-1.)) ;
#10844=DIRECTION('ref_axis',(1.,0.,0.)) ;
#10845=DIRECTION('',(0.857167300702109,1.04972719113861E-16,0.51503807491006)) ;
#10846=DIRECTION('center_axis',(0.,0.,-1.)) ;
#10847=DIRECTION('ref_axis',(1.,0.,0.)) ;
#10848=DIRECTION('',(0.857167300702111,1.04972719113862E-16,0.515038074910057)) ;
#10849=DIRECTION('center_axis',(0.,0.,-1.)) ;
#10850=DIRECTION('ref_axis',(1.,0.,0.)) ;
#10851=DIRECTION('',(0.857167300702109,1.04972719113861E-16,0.51503807491006)) ;
#10852=DIRECTION('center_axis',(0.,0.,-1.)) ;
#10853=DIRECTION('ref_axis',(1.,0.,0.)) ;
#10854=DIRECTION('',(0.857167300702111,1.04972719113862E-16,0.515038074910057)) ;
#10855=DIRECTION('center_axis',(0.,0.,-1.)) ;
#10856=DIRECTION('ref_axis',(-1.,1.25569625557165E-14,0.)) ;
#10857=DIRECTION('center_axis',(0.,1.,0.)) ;
#10858=DIRECTION('ref_axis',(1.,0.,0.)) ;
#10859=DIRECTION('center_axis',(0.,1.,0.)) ;
#10860=DIRECTION('ref_axis',(1.,0.,0.)) ;
#10861=DIRECTION('',(0.,1.,0.)) ;
#10862=DIRECTION('center_axis',(0.,-1.,0.)) ;
#10863=DIRECTION('ref_axis',(1.,0.,0.)) ;
#10864=DIRECTION('center_axis',(0.,0.,-1.)) ;
#10865=DIRECTION('ref_axis',(1.,0.,0.)) ;
#10866=DIRECTION('',(0.857167300702113,1.04972719113862E-16,0.515038074910054)) ;
#10867=DIRECTION('center_axis',(0.,0.,-1.)) ;
#10868=DIRECTION('ref_axis',(-1.,-1.2312033195887E-14,0.)) ;
#10869=DIRECTION('center_axis',(0.,1.,0.)) ;
#10870=DIRECTION('ref_axis',(1.,0.,0.)) ;
#10871=DIRECTION('center_axis',(0.,1.,0.)) ;
#10872=DIRECTION('ref_axis',(1.,0.,0.)) ;
#10873=DIRECTION('',(0.,1.,0.)) ;
#10874=DIRECTION('center_axis',(0.,-1.,0.)) ;
#10875=DIRECTION('ref_axis',(1.,0.,0.)) ;
#10876=DIRECTION('center_axis',(0.,0.,-1.)) ;
#10877=DIRECTION('ref_axis',(1.,0.,0.)) ;
#10878=DIRECTION('',(0.857167300702113,1.04972719113862E-16,0.515038074910054)) ;
#10879=DIRECTION('center_axis',(-1.,0.,0.)) ;
#10880=DIRECTION('ref_axis',(0.,0.,-1.)) ;
#10881=DIRECTION('',(-1.,0.,0.)) ;
#10882=DIRECTION('center_axis',(0.,0.,-1.)) ;
#10883=DIRECTION('ref_axis',(1.,0.,0.)) ;
#10884=DIRECTION('center_axis',(0.,0.,-1.)) ;
#10885=DIRECTION('ref_axis',(1.,0.,0.)) ;
#10886=DIRECTION('',(0.,0.,-1.)) ;
#10887=DIRECTION('center_axis',(0.,0.,-1.)) ;
#10888=DIRECTION('ref_axis',(1.,0.,0.)) ;
#10889=DIRECTION('center_axis',(0.,0.,1.)) ;
#10890=DIRECTION('ref_axis',(1.,0.,0.)) ;
#10891=DIRECTION('center_axis',(-1.,0.,0.)) ;
#10892=DIRECTION('ref_axis',(0.,0.,-1.)) ;
#10893=DIRECTION('',(-1.,0.,0.)) ;
#10894=DIRECTION('center_axis',(0.,0.,-1.)) ;
#10895=DIRECTION('ref_axis',(1.,0.,0.)) ;
#10896=DIRECTION('center_axis',(0.,0.,-1.)) ;
#10897=DIRECTION('ref_axis',(1.,0.,0.)) ;
#10898=DIRECTION('',(0.,0.,-1.)) ;
#10899=DIRECTION('center_axis',(0.,0.,-1.)) ;
#10900=DIRECTION('ref_axis',(1.,0.,0.)) ;
#10901=DIRECTION('center_axis',(0.,0.,1.)) ;
#10902=DIRECTION('ref_axis',(1.,0.,0.)) ;
#10903=DIRECTION('center_axis',(0.,1.,0.)) ;
#10904=DIRECTION('ref_axis',(1.,0.,0.)) ;
#10905=DIRECTION('center_axis',(0.,1.,0.)) ;
#10906=DIRECTION('ref_axis',(1.,0.,0.)) ;
#10907=DIRECTION('',(0.,1.,0.)) ;
#10908=DIRECTION('center_axis',(0.,-1.,0.)) ;
#10909=DIRECTION('ref_axis',(1.,0.,0.)) ;
#10910=DIRECTION('center_axis',(0.,1.,0.)) ;
#10911=DIRECTION('ref_axis',(1.,0.,0.)) ;
#10912=DIRECTION('center_axis',(0.,1.,0.)) ;
#10913=DIRECTION('ref_axis',(1.,0.,0.)) ;
#10914=DIRECTION('',(0.,1.,0.)) ;
#10915=DIRECTION('center_axis',(0.,-1.,0.)) ;
#10916=DIRECTION('ref_axis',(1.,0.,0.)) ;
#10917=DIRECTION('center_axis',(0.,1.,0.)) ;
#10918=DIRECTION('ref_axis',(1.,0.,0.)) ;
#10919=DIRECTION('',(0.,-1.,0.)) ;
#10920=DIRECTION('center_axis',(0.,-1.,0.)) ;
#10921=DIRECTION('ref_axis',(1.,0.,0.)) ;
#10922=DIRECTION('',(0.,1.,0.)) ;
#10923=DIRECTION('center_axis',(0.,1.,0.)) ;
#10924=DIRECTION('ref_axis',(1.,0.,0.)) ;
#10925=DIRECTION('center_axis',(0.,1.,0.)) ;
#10926=DIRECTION('ref_axis',(1.,0.,0.)) ;
#10927=DIRECTION('',(0.,-1.,0.)) ;
#10928=DIRECTION('center_axis',(0.,-1.,0.)) ;
#10929=DIRECTION('ref_axis',(1.,0.,0.)) ;
#10930=DIRECTION('',(0.,1.,0.)) ;
#10931=DIRECTION('center_axis',(0.,1.,0.)) ;
#10932=DIRECTION('ref_axis',(1.,0.,0.)) ;
#10933=DIRECTION('center_axis',(-1.,0.,0.)) ;
#10934=DIRECTION('ref_axis',(0.,0.,1.)) ;
#10935=DIRECTION('',(0.,0.,1.)) ;
#10936=DIRECTION('',(0.,1.,0.)) ;
#10937=DIRECTION('',(0.,0.,1.)) ;
#10938=DIRECTION('center_axis',(0.,1.,0.)) ;
#10939=DIRECTION('ref_axis',(1.,0.,0.)) ;
#10940=DIRECTION('center_axis',(0.,1.,0.)) ;
#10941=DIRECTION('ref_axis',(-1.,0.,0.)) ;
#10942=DIRECTION('',(1.,0.,0.)) ;
#10943=DIRECTION('',(0.,0.,1.)) ;
#10944=DIRECTION('',(-1.,0.,0.)) ;
#10945=DIRECTION('center_axis',(-1.,0.,0.)) ;
#10946=DIRECTION('ref_axis',(0.,0.,1.)) ;
#10947=DIRECTION('',(0.,0.,1.)) ;
#10948=DIRECTION('',(0.,1.,0.)) ;
#10949=DIRECTION('',(0.,0.,1.)) ;
#10950=DIRECTION('center_axis',(0.,1.,0.)) ;
#10951=DIRECTION('ref_axis',(1.,0.,0.)) ;
#10952=DIRECTION('center_axis',(0.,1.,0.)) ;
#10953=DIRECTION('ref_axis',(-1.,0.,0.)) ;
#10954=DIRECTION('',(1.,0.,0.)) ;
#10955=DIRECTION('',(0.,0.,1.)) ;
#10956=DIRECTION('',(-1.,0.,0.)) ;
#10957=DIRECTION('center_axis',(0.,0.707106781186548,0.707106781186548)) ;
#10958=DIRECTION('ref_axis',(1.,0.,0.)) ;
#10959=DIRECTION('',(0.,-0.707106781186548,0.707106781186548)) ;
#10960=DIRECTION('',(1.,0.,0.)) ;
#10961=DIRECTION('',(0.,0.707106781186548,-0.707106781186548)) ;
#10962=DIRECTION('',(-1.,0.,0.)) ;
#10963=DIRECTION('center_axis',(0.,1.,0.)) ;
#10964=DIRECTION('ref_axis',(-1.,0.,0.)) ;
#10965=DIRECTION('',(0.,0.,1.)) ;
#10966=DIRECTION('',(-1.,0.,0.)) ;
#10967=DIRECTION('',(-1.,0.,0.)) ;
#10968=DIRECTION('',(-1.,0.,0.)) ;
#10969=DIRECTION('',(0.,0.,1.)) ;
#10970=DIRECTION('center_axis',(1.,0.,0.)) ;
#10971=DIRECTION('ref_axis',(0.,1.,0.)) ;
#10972=DIRECTION('',(0.,1.,0.)) ;
#10973=DIRECTION('',(0.,0.,-1.)) ;
#10974=DIRECTION('',(0.,-1.,0.)) ;
#10975=DIRECTION('',(0.,0.,1.)) ;
#10976=DIRECTION('',(0.,1.,0.)) ;
#10977=DIRECTION('',(0.,0.,-1.)) ;
#10978=DIRECTION('',(0.,-1.,0.)) ;
#10979=DIRECTION('',(0.,0.,1.)) ;
#10980=DIRECTION('',(0.,1.,0.)) ;
#10981=DIRECTION('',(0.,0.707106781186548,0.707106781186548)) ;
#10982=DIRECTION('',(0.,0.,1.)) ;
#10983=DIRECTION('',(0.,1.,0.)) ;
#10984=DIRECTION('',(0.,0.,1.)) ;
#10985=DIRECTION('',(0.,0.,1.)) ;
#10986=DIRECTION('',(0.,1.,0.)) ;
#10987=DIRECTION('',(0.,0.,1.)) ;
#10988=DIRECTION('',(0.,0.,1.)) ;
#10989=DIRECTION('',(0.,1.,0.)) ;
#10990=DIRECTION('center_axis',(0.,-0.707106781186548,0.707106781186548)) ;
#10991=DIRECTION('ref_axis',(1.,0.,0.)) ;
#10992=DIRECTION('',(-1.,0.,0.)) ;
#10993=DIRECTION('',(0.,-0.707106781186548,-0.707106781186548)) ;
#10994=DIRECTION('',(1.,0.,0.)) ;
#10995=DIRECTION('center_axis',(0.,-1.,0.)) ;
#10996=DIRECTION('ref_axis',(1.,0.,0.)) ;
#10997=DIRECTION('',(0.,0.,1.)) ;
#10998=DIRECTION('',(1.,0.,0.)) ;
#10999=DIRECTION('',(1.,0.,0.)) ;
#11000=DIRECTION('',(1.,0.,0.)) ;
#11001=DIRECTION('center_axis',(0.,0.,1.)) ;
#11002=DIRECTION('ref_axis',(1.,0.,0.)) ;
#11003=DIRECTION('center_axis',(0.,0.,1.)) ;
#11004=DIRECTION('ref_axis',(1.,0.,0.)) ;
#11005=DIRECTION('',(0.,0.,-1.)) ;
#11006=DIRECTION('center_axis',(0.,0.,1.)) ;
#11007=DIRECTION('ref_axis',(1.,0.,0.)) ;
#11008=DIRECTION('',(0.,0.,-1.)) ;
#11009=DIRECTION('center_axis',(0.,0.,-1.)) ;
#11010=DIRECTION('ref_axis',(1.,0.,0.)) ;
#11011=DIRECTION('center_axis',(0.,0.,1.)) ;
#11012=DIRECTION('ref_axis',(1.,0.,0.)) ;
#11013=DIRECTION('center_axis',(0.,0.,-1.)) ;
#11014=DIRECTION('ref_axis',(1.,0.,0.)) ;
#11015=DIRECTION('',(0.,0.,1.)) ;
#11016=DIRECTION('center_axis',(0.,0.,1.)) ;
#11017=DIRECTION('ref_axis',(1.,0.,0.)) ;
#11018=DIRECTION('center_axis',(0.,0.,-1.)) ;
#11019=DIRECTION('ref_axis',(-1.,0.,0.)) ;
#11020=DIRECTION('center_axis',(0.,0.,-1.)) ;
#11021=DIRECTION('ref_axis',(-1.,0.,0.)) ;
#11022=DIRECTION('',(0.,1.,0.)) ;
#11023=DIRECTION('center_axis',(0.,0.,1.)) ;
#11024=DIRECTION('ref_axis',(1.,0.,0.)) ;
#11025=DIRECTION('center_axis',(-1.,0.,0.)) ;
#11026=DIRECTION('ref_axis',(0.,-1.,0.)) ;
#11027=DIRECTION('',(0.,-1.,0.)) ;
#11028=DIRECTION('',(0.,0.,-1.)) ;
#11029=DIRECTION('',(0.,1.,0.)) ;
#11030=DIRECTION('',(0.,0.,1.)) ;
#11031=DIRECTION('',(0.,-1.,0.)) ;
#11032=DIRECTION('',(0.,0.,1.)) ;
#11033=DIRECTION('',(0.,-1.,0.)) ;
#11034=DIRECTION('',(0.,-1.,0.)) ;
#11035=DIRECTION('',(0.,-1.,0.)) ;
#11036=DIRECTION('',(0.,0.,-1.)) ;
#11037=DIRECTION('',(0.,-1.,0.)) ;
#11038=DIRECTION('',(0.,-1.,0.)) ;
#11039=DIRECTION('',(0.,0.,-1.)) ;
#11040=DIRECTION('',(0.,1.,0.)) ;
#11041=DIRECTION('',(0.,-1.,0.)) ;
#11042=DIRECTION('',(0.,0.,-1.)) ;
#11043=DIRECTION('',(0.,1.,0.)) ;
#11044=DIRECTION('center_axis',(0.,0.,1.)) ;
#11045=DIRECTION('ref_axis',(1.,0.,0.)) ;
#11046=DIRECTION('center_axis',(0.,0.,-1.)) ;
#11047=DIRECTION('ref_axis',(1.,0.,0.)) ;
#11048=DIRECTION('center_axis',(0.,0.,-1.)) ;
#11049=DIRECTION('ref_axis',(-1.,0.,0.)) ;
#11050=DIRECTION('',(-1.,0.,0.)) ;
#11051=DIRECTION('center_axis',(0.,0.,1.)) ;
#11052=DIRECTION('ref_axis',(1.,0.,0.)) ;
#11053=DIRECTION('',(1.,0.,0.)) ;
#11054=DIRECTION('',(0.,1.,0.)) ;
#11055=DIRECTION('center_axis',(0.,1.,0.)) ;
#11056=DIRECTION('ref_axis',(-1.,0.,0.)) ;
#11057=DIRECTION('center_axis',(0.,1.,0.)) ;
#11058=DIRECTION('ref_axis',(-1.,0.,0.)) ;
#11059=DIRECTION('center_axis',(0.,1.,0.)) ;
#11060=DIRECTION('ref_axis',(1.,0.,0.)) ;
#11061=DIRECTION('center_axis',(0.,0.,1.)) ;
#11062=DIRECTION('ref_axis',(1.,0.,0.)) ;
#11063=DIRECTION('',(0.,1.,0.)) ;
#11064=DIRECTION('',(-1.,0.,0.)) ;
#11065=DIRECTION('',(0.,1.,0.)) ;
#11066=DIRECTION('',(-1.,0.,0.)) ;
#11067=DIRECTION('center_axis',(0.,1.,0.)) ;
#11068=DIRECTION('ref_axis',(-1.,0.,0.)) ;
#11069=DIRECTION('',(0.,0.,-1.)) ;
#11070=DIRECTION('',(0.,0.,1.)) ;
#11071=DIRECTION('',(-1.,0.,0.)) ;
#11072=DIRECTION('center_axis',(1.,0.,0.)) ;
#11073=DIRECTION('ref_axis',(0.,1.,0.)) ;
#11074=DIRECTION('',(0.,1.,0.)) ;
#11075=DIRECTION('',(0.,0.,1.)) ;
#11076=DIRECTION('center_axis',(0.,0.,1.)) ;
#11077=DIRECTION('ref_axis',(1.,0.,0.)) ;
#11078=DIRECTION('center_axis',(0.,0.,1.)) ;
#11079=DIRECTION('ref_axis',(1.,0.,0.)) ;
#11080=DIRECTION('',(0.,0.,-1.)) ;
#11081=DIRECTION('center_axis',(0.,0.,1.)) ;
#11082=DIRECTION('ref_axis',(1.,0.,0.)) ;
#11083=DIRECTION('center_axis',(0.,0.,1.)) ;
#11084=DIRECTION('ref_axis',(1.,0.,0.)) ;
#11085=DIRECTION('center_axis',(0.,0.,-1.)) ;
#11086=DIRECTION('ref_axis',(1.,0.,0.)) ;
#11087=DIRECTION('center_axis',(0.,0.,1.)) ;
#11088=DIRECTION('ref_axis',(1.,0.,0.)) ;
#11089=DIRECTION('center_axis',(0.,0.,-1.)) ;
#11090=DIRECTION('ref_axis',(-1.,0.,0.)) ;
#11091=DIRECTION('center_axis',(0.,0.,-1.)) ;
#11092=DIRECTION('ref_axis',(-1.,0.,0.)) ;
#11093=DIRECTION('center_axis',(0.,0.,1.)) ;
#11094=DIRECTION('ref_axis',(1.,0.,0.)) ;
#11095=DIRECTION('center_axis',(0.,0.,-1.)) ;
#11096=DIRECTION('ref_axis',(-1.,0.,0.)) ;
#11097=DIRECTION('',(-1.,0.,0.)) ;
#11098=DIRECTION('center_axis',(0.,0.,1.)) ;
#11099=DIRECTION('ref_axis',(1.,0.,0.)) ;
#11100=DIRECTION('',(1.,0.,0.)) ;
#11101=DIRECTION('',(0.,1.,0.)) ;
#11102=DIRECTION('center_axis',(0.,1.,0.)) ;
#11103=DIRECTION('ref_axis',(-1.,0.,0.)) ;
#11104=DIRECTION('center_axis',(0.,1.,0.)) ;
#11105=DIRECTION('ref_axis',(-1.,0.,0.)) ;
#11106=DIRECTION('center_axis',(0.,1.,0.)) ;
#11107=DIRECTION('ref_axis',(1.,0.,0.)) ;
#11108=DIRECTION('center_axis',(0.,0.,1.)) ;
#11109=DIRECTION('ref_axis',(1.,0.,0.)) ;
#11110=DIRECTION('',(0.,1.,0.)) ;
#11111=DIRECTION('',(1.,0.,0.)) ;
#11112=DIRECTION('',(0.,1.,0.)) ;
#11113=DIRECTION('',(1.,0.,0.)) ;
#11114=DIRECTION('center_axis',(0.,-1.,0.)) ;
#11115=DIRECTION('ref_axis',(1.,0.,0.)) ;
#11116=DIRECTION('',(0.,0.,1.)) ;
#11117=DIRECTION('',(1.,0.,0.)) ;
#11118=DIRECTION('',(0.,0.,1.)) ;
#11119=DIRECTION('center_axis',(1.,0.,0.)) ;
#11120=DIRECTION('ref_axis',(0.,1.,0.)) ;
#11121=DIRECTION('',(0.,1.,0.)) ;
#11122=DIRECTION('',(0.,0.,-1.)) ;
#11123=DIRECTION('center_axis',(0.,0.,1.)) ;
#11124=DIRECTION('ref_axis',(1.,0.,0.)) ;
#11125=DIRECTION('',(0.,-1.,0.)) ;
#11126=DIRECTION('',(1.,0.,0.)) ;
#11127=DIRECTION('',(0.,1.,0.)) ;
#11128=DIRECTION('center_axis',(0.,1.,0.)) ;
#11129=DIRECTION('ref_axis',(-1.,0.,0.)) ;
#11130=DIRECTION('',(0.,0.,1.)) ;
#11131=DIRECTION('',(-1.,0.,0.)) ;
#11132=DIRECTION('',(0.,0.,1.)) ;
#11133=DIRECTION('center_axis',(1.,0.,0.)) ;
#11134=DIRECTION('ref_axis',(0.,1.,0.)) ;
#11135=DIRECTION('',(0.,1.,0.)) ;
#11136=DIRECTION('',(0.,0.,1.)) ;
#11137=DIRECTION('center_axis',(0.,-1.,0.)) ;
#11138=DIRECTION('ref_axis',(1.,0.,0.)) ;
#11139=DIRECTION('',(0.,0.,1.)) ;
#11140=DIRECTION('center_axis',(0.,0.,1.)) ;
#11141=DIRECTION('ref_axis',(1.,0.,0.)) ;
#11142=DIRECTION('',(0.,1.,0.)) ;
#11143=DIRECTION('',(-1.,0.,0.)) ;
#11144=DIRECTION('',(0.,-1.,0.)) ;
#11145=DIRECTION('center_axis',(0.,1.,0.)) ;
#11146=DIRECTION('ref_axis',(-1.,0.,0.)) ;
#11147=DIRECTION('',(0.,0.,1.)) ;
#11148=DIRECTION('',(0.,0.,1.)) ;
#11149=DIRECTION('center_axis',(1.,0.,0.)) ;
#11150=DIRECTION('ref_axis',(0.,1.,0.)) ;
#11151=DIRECTION('',(0.,1.,0.)) ;
#11152=DIRECTION('',(0.,0.,1.)) ;
#11153=DIRECTION('center_axis',(0.,-1.,0.)) ;
#11154=DIRECTION('ref_axis',(1.,0.,0.)) ;
#11155=DIRECTION('',(1.,0.,0.)) ;
#11156=DIRECTION('',(0.,0.,1.)) ;
#11157=DIRECTION('center_axis',(0.,0.,1.)) ;
#11158=DIRECTION('ref_axis',(1.,0.,0.)) ;
#11159=DIRECTION('',(0.,-1.,0.)) ;
#11160=DIRECTION('',(0.,-1.,0.)) ;
#11161=DIRECTION('',(1.,0.,0.)) ;
#11162=DIRECTION('',(0.,1.,0.)) ;
#11163=DIRECTION('',(-1.,0.,0.)) ;
#11164=DIRECTION('',(0.,-1.,0.)) ;
#11165=DIRECTION('center_axis',(1.,0.,0.)) ;
#11166=DIRECTION('ref_axis',(0.,1.,0.)) ;
#11167=DIRECTION('',(0.,0.,-1.)) ;
#11168=DIRECTION('',(0.,1.,0.)) ;
#11169=DIRECTION('',(0.,0.,1.)) ;
#11170=DIRECTION('center_axis',(0.,-1.,0.)) ;
#11171=DIRECTION('ref_axis',(1.,0.,0.)) ;
#11172=DIRECTION('',(1.,0.,0.)) ;
#11173=DIRECTION('',(1.,0.,0.)) ;
#11174=DIRECTION('center_axis',(0.,0.,1.)) ;
#11175=DIRECTION('ref_axis',(1.,0.,0.)) ;
#11176=DIRECTION('',(0.,-1.,0.)) ;
#11177=DIRECTION('',(1.,0.,0.)) ;
#11178=DIRECTION('center_axis',(0.,1.,0.)) ;
#11179=DIRECTION('ref_axis',(-1.,0.,0.)) ;
#11180=DIRECTION('',(0.,0.,1.)) ;
#11181=DIRECTION('',(-1.,0.,0.)) ;
#11182=DIRECTION('',(-1.,0.,0.)) ;
#11183=DIRECTION('center_axis',(0.,-1.,0.)) ;
#11184=DIRECTION('ref_axis',(1.,0.,0.)) ;
#11185=DIRECTION('',(0.,0.,1.)) ;
#11186=DIRECTION('center_axis',(-1.,0.,0.)) ;
#11187=DIRECTION('ref_axis',(0.,-1.,0.)) ;
#11188=DIRECTION('',(0.,-1.,0.)) ;
#11189=DIRECTION('center_axis',(0.,0.,1.)) ;
#11190=DIRECTION('ref_axis',(1.,0.,0.)) ;
#11191=DIRECTION('',(-1.,0.,0.)) ;
#11192=DIRECTION('center_axis',(0.,0.,1.)) ;
#11193=DIRECTION('ref_axis',(1.,0.,0.)) ;
#11194=DIRECTION('',(1.,0.,0.)) ;
#11195=DIRECTION('center_axis',(0.,0.,1.)) ;
#11196=DIRECTION('ref_axis',(1.,0.,0.)) ;
#11197=DIRECTION('',(-1.,0.,0.)) ;
#11198=DIRECTION('',(0.,-1.,0.)) ;
#11199=DIRECTION('center_axis',(0.,0.,1.)) ;
#11200=DIRECTION('ref_axis',(1.,0.,0.)) ;
#11201=DIRECTION('',(0.,-1.,0.)) ;
#11202=DIRECTION('',(1.,0.,0.)) ;
#11203=DIRECTION('center_axis',(0.,1.,0.)) ;
#11204=DIRECTION('ref_axis',(-1.,0.,0.)) ;
#11205=DIRECTION('',(0.,0.,1.)) ;
#11206=DIRECTION('center_axis',(0.,-1.,0.)) ;
#11207=DIRECTION('ref_axis',(1.,0.,0.)) ;
#11208=DIRECTION('',(0.,0.,1.)) ;
#11209=DIRECTION('center_axis',(-1.,0.,0.)) ;
#11210=DIRECTION('ref_axis',(0.,-1.,0.)) ;
#11211=DIRECTION('center_axis',(0.,1.,0.)) ;
#11212=DIRECTION('ref_axis',(-1.,0.,0.)) ;
#11213=DIRECTION('',(-1.,0.,0.)) ;
#11214=DIRECTION('center_axis',(-1.,0.,0.)) ;
#11215=DIRECTION('ref_axis',(0.,-1.,0.)) ;
#11216=DIRECTION('',(0.,-1.,0.)) ;
#11217=DIRECTION('center_axis',(0.,0.,1.)) ;
#11218=DIRECTION('ref_axis',(1.,0.,0.)) ;
#13423=CARTESIAN_POINT('',(0.,0.,0.)) ;
#13424=CARTESIAN_POINT('Origin',(-84.75,-52.3,27.675)) ;
#13425=CARTESIAN_POINT('',(-85.95,-52.3,27.6)) ;
#13426=CARTESIAN_POINT('Origin',(-84.75,-52.3,27.6)) ;
#13427=CARTESIAN_POINT('',(-85.8,-52.3,27.75)) ;
#13428=CARTESIAN_POINT('',(-85.875,-52.3,27.675)) ;
#13429=CARTESIAN_POINT('Origin',(-84.75,-52.3,27.75)) ;
#13430=CARTESIAN_POINT('Origin',(-78.25,-52.3,27.6)) ;
#13431=CARTESIAN_POINT('',(-87.25,-45.3,27.6)) ;
#13432=CARTESIAN_POINT('',(-87.25,-59.3,27.6)) ;
#13433=CARTESIAN_POINT('',(-87.25,-45.3,27.6)) ;
#13434=CARTESIAN_POINT('',(-69.25,-45.3,27.6)) ;
#13435=CARTESIAN_POINT('',(-69.25,-45.3,27.6)) ;
#13436=CARTESIAN_POINT('',(-69.25,-59.3,27.6)) ;
#13437=CARTESIAN_POINT('',(-69.25,-59.3,27.6)) ;
#13438=CARTESIAN_POINT('',(-87.25,-59.3,27.6)) ;
#13439=CARTESIAN_POINT('',(-72.95,-52.3,27.6)) ;
#13440=CARTESIAN_POINT('Origin',(-71.75,-52.3,27.6)) ;
#13441=CARTESIAN_POINT('Origin',(-84.75,-52.3,27.6)) ;
#13442=CARTESIAN_POINT('',(-85.8,-52.3,33.4)) ;
#13443=CARTESIAN_POINT('',(-85.8,-52.3,27.6)) ;
#13444=CARTESIAN_POINT('Origin',(-84.75,-52.3,33.4)) ;
#13445=CARTESIAN_POINT('Origin',(-84.75,52.3,27.675)) ;
#13446=CARTESIAN_POINT('',(-85.95,52.3,27.6)) ;
#13447=CARTESIAN_POINT('Origin',(-84.75,52.3,27.6)) ;
#13448=CARTESIAN_POINT('',(-85.8,52.3,27.75)) ;
#13449=CARTESIAN_POINT('',(-85.875,52.3,27.675)) ;
#13450=CARTESIAN_POINT('Origin',(-84.75,52.3,27.75)) ;
#13451=CARTESIAN_POINT('Origin',(-78.25,52.3,27.6)) ;
#13452=CARTESIAN_POINT('',(-87.25,59.3,27.6)) ;
#13453=CARTESIAN_POINT('',(-87.25,45.3,27.6)) ;
#13454=CARTESIAN_POINT('',(-87.25,59.3,27.6)) ;
#13455=CARTESIAN_POINT('',(-69.25,59.3,27.6)) ;
#13456=CARTESIAN_POINT('',(-69.25,59.3,27.6)) ;
#13457=CARTESIAN_POINT('',(-69.25,45.3,27.6)) ;
#13458=CARTESIAN_POINT('',(-69.25,45.3,27.6)) ;
#13459=CARTESIAN_POINT('',(-87.25,45.3,27.6)) ;
#13460=CARTESIAN_POINT('',(-72.95,52.3,27.6)) ;
#13461=CARTESIAN_POINT('Origin',(-71.75,52.3,27.6)) ;
#13462=CARTESIAN_POINT('Origin',(-84.75,52.3,27.6)) ;
#13463=CARTESIAN_POINT('',(-85.8,52.3,33.4)) ;
#13464=CARTESIAN_POINT('',(-85.8,52.3,27.6)) ;
#13465=CARTESIAN_POINT('Origin',(-84.75,52.3,33.4)) ;
#13466=CARTESIAN_POINT('Origin',(84.75,52.3,27.675)) ;
#13467=CARTESIAN_POINT('',(83.55,52.3,27.6)) ;
#13468=CARTESIAN_POINT('Origin',(84.75,52.3,27.6)) ;
#13469=CARTESIAN_POINT('',(83.7,52.3,27.75)) ;
#13470=CARTESIAN_POINT('',(83.625,52.3,27.675)) ;
#13471=CARTESIAN_POINT('Origin',(84.75,52.3,27.75)) ;
#13472=CARTESIAN_POINT('Origin',(78.25,52.3,27.6)) ;
#13473=CARTESIAN_POINT('',(69.25,59.3,27.6)) ;
#13474=CARTESIAN_POINT('',(69.25,45.3,27.6)) ;
#13475=CARTESIAN_POINT('',(69.25,59.3,27.6)) ;
#13476=CARTESIAN_POINT('',(87.25,59.3,27.6)) ;
#13477=CARTESIAN_POINT('',(87.25,59.3,27.6)) ;
#13478=CARTESIAN_POINT('',(87.25,45.3,27.6)) ;
#13479=CARTESIAN_POINT('',(87.25,45.3,27.6)) ;
#13480=CARTESIAN_POINT('',(69.25,45.3,27.6)) ;
#13481=CARTESIAN_POINT('',(70.55,52.3,27.6)) ;
#13482=CARTESIAN_POINT('Origin',(71.75,52.3,27.6)) ;
#13483=CARTESIAN_POINT('Origin',(84.75,52.3,27.6)) ;
#13484=CARTESIAN_POINT('',(83.7,52.3,33.4)) ;
#13485=CARTESIAN_POINT('',(83.7,52.3,27.6)) ;
#13486=CARTESIAN_POINT('Origin',(84.75,52.3,33.4)) ;
#13487=CARTESIAN_POINT('Origin',(84.75,-52.3,27.675)) ;
#13488=CARTESIAN_POINT('',(83.55,-52.3,27.6)) ;
#13489=CARTESIAN_POINT('Origin',(84.75,-52.3,27.6)) ;
#13490=CARTESIAN_POINT('',(83.7,-52.3,27.75)) ;
#13491=CARTESIAN_POINT('',(83.625,-52.3,27.675)) ;
#13492=CARTESIAN_POINT('Origin',(84.75,-52.3,27.75)) ;
#13493=CARTESIAN_POINT('Origin',(78.25,-52.3,27.6)) ;
#13494=CARTESIAN_POINT('',(69.25,-45.3,27.6)) ;
#13495=CARTESIAN_POINT('',(69.25,-59.3,27.6)) ;
#13496=CARTESIAN_POINT('',(69.25,-45.3,27.6)) ;
#13497=CARTESIAN_POINT('',(87.25,-45.3,27.6)) ;
#13498=CARTESIAN_POINT('',(87.25,-45.3,27.6)) ;
#13499=CARTESIAN_POINT('',(87.25,-59.3,27.6)) ;
#13500=CARTESIAN_POINT('',(87.25,-59.3,27.6)) ;
#13501=CARTESIAN_POINT('',(69.25,-59.3,27.6)) ;
#13502=CARTESIAN_POINT('',(70.55,-52.3,27.6)) ;
#13503=CARTESIAN_POINT('Origin',(71.75,-52.3,27.6)) ;
#13504=CARTESIAN_POINT('Origin',(84.75,-52.3,27.6)) ;
#13505=CARTESIAN_POINT('',(83.7,-52.3,33.4)) ;
#13506=CARTESIAN_POINT('',(83.7,-52.3,27.6)) ;
#13507=CARTESIAN_POINT('Origin',(84.75,-52.3,33.4)) ;
#13508=CARTESIAN_POINT('Origin',(71.75,52.3,27.675)) ;
#13509=CARTESIAN_POINT('',(70.7,52.3,27.75)) ;
#13510=CARTESIAN_POINT('',(70.625,52.3,27.675)) ;
#13511=CARTESIAN_POINT('Origin',(71.75,52.3,27.75)) ;
#13512=CARTESIAN_POINT('Origin',(71.75,52.3,27.6)) ;
#13513=CARTESIAN_POINT('',(70.7,52.3,33.4)) ;
#13514=CARTESIAN_POINT('',(70.7,52.3,27.6)) ;
#13515=CARTESIAN_POINT('',(70.7183994382024,52.1042954244305,33.4)) ;
#13516=CARTESIAN_POINT('Origin',(71.75,52.3,33.4)) ;
#13517=CARTESIAN_POINT('',(70.7183994382024,52.4957045755694,33.4)) ;
#13518=CARTESIAN_POINT('Ctrl Pts',(70.7183994382024,52.4957045755694,33.4)) ;
#13519=CARTESIAN_POINT('Ctrl Pts',(70.7319761095756,52.5672701062946,33.389125081463)) ;
#13520=CARTESIAN_POINT('Ctrl Pts',(70.7531407522362,52.6376371859408,33.3724123738805)) ;
#13521=CARTESIAN_POINT('Ctrl Pts',(70.8341056071048,52.8316627295715,33.3125298347947)) ;
#13522=CARTESIAN_POINT('Ctrl Pts',(70.9124422905779,52.9458062688949,33.2592888082397)) ;
#13523=CARTESIAN_POINT('Ctrl Pts',(71.0924279408069,53.128845249026,33.1588871128703)) ;
#13524=CARTESIAN_POINT('Ctrl Pts',(71.2082663884949,53.2104458534536,33.1040987390693)) ;
#13525=CARTESIAN_POINT('Ctrl Pts',(71.4676871756213,53.3211202136295,33.0155789759107)) ;
#13526=CARTESIAN_POINT('Ctrl Pts',(71.611512060708,53.35,32.98231678229)) ;
#13527=CARTESIAN_POINT('Ctrl Pts',(71.8811502184983,53.35,32.9491868010911)) ;
#13528=CARTESIAN_POINT('Ctrl Pts',(72.021484418179,53.3238190465072,32.9460485518659)) ;
#13529=CARTESIAN_POINT('Ctrl Pts',(72.2790771456966,53.2175982662943,32.9649830273315)) ;
#13530=CARTESIAN_POINT('Ctrl Pts',(72.3964053699774,53.1376182539018,32.9864379744825)) ;
#13531=CARTESIAN_POINT('Ctrl Pts',(72.5827722667432,52.9530317340365,33.0322038118174)) ;
#13532=CARTESIAN_POINT('Ctrl Pts',(72.6641459041156,52.835355369045,33.0596974322278)) ;
#13533=CARTESIAN_POINT('Ctrl Pts',(72.7727880560022,52.5759934056159,33.1003519438363)) ;
#13534=CARTESIAN_POINT('Ctrl Pts',(72.8,52.4341327809988,33.1125413911823)) ;
#13535=CARTESIAN_POINT('Ctrl Pts',(72.8,52.3,33.1125413911823)) ;
#13536=CARTESIAN_POINT('Ctrl Pts',(72.8,52.1658672190012,33.1125413911823)) ;
#13537=CARTESIAN_POINT('Ctrl Pts',(72.7727880560022,52.0240065943841,33.1003519438363)) ;
#13538=CARTESIAN_POINT('Ctrl Pts',(72.6641459041156,51.764644630955,33.0596974322278)) ;
#13539=CARTESIAN_POINT('Ctrl Pts',(72.5827722667432,51.6469682659635,33.0322038118174)) ;
#13540=CARTESIAN_POINT('Ctrl Pts',(72.3964053699774,51.4623817460982,32.9864379744825)) ;
#13541=CARTESIAN_POINT('Ctrl Pts',(72.2790771456966,51.3824017337057,32.9649830273315)) ;
#13542=CARTESIAN_POINT('Ctrl Pts',(72.021484418179,51.2761809534928,32.9460485518659)) ;
#13543=CARTESIAN_POINT('Ctrl Pts',(71.8811502184983,51.25,32.9491868010911)) ;
#13544=CARTESIAN_POINT('Ctrl Pts',(71.611512060708,51.25,32.98231678229)) ;
#13545=CARTESIAN_POINT('Ctrl Pts',(71.4676871756213,51.2788797863705,33.0155789759107)) ;
#13546=CARTESIAN_POINT('Ctrl Pts',(71.2082663884949,51.3895541465464,33.1040987390693)) ;
#13547=CARTESIAN_POINT('Ctrl Pts',(71.0924279408069,51.471154750974,33.1588871128703)) ;
#13548=CARTESIAN_POINT('Ctrl Pts',(70.9124422905779,51.6541937311051,33.2592888082397)) ;
#13549=CARTESIAN_POINT('Ctrl Pts',(70.8341056071048,51.7683372704285,33.3125298347947)) ;
#13550=CARTESIAN_POINT('Ctrl Pts',(70.7531407522363,51.9623628140592,33.3724123738805)) ;
#13551=CARTESIAN_POINT('Ctrl Pts',(70.7319761095756,52.0327298937054,33.389125081463)) ;
#13552=CARTESIAN_POINT('Ctrl Pts',(70.7183994382024,52.1042954244305,33.4)) ;
#13553=CARTESIAN_POINT('Origin',(71.75,52.3,33.4)) ;
#13554=CARTESIAN_POINT('Origin',(71.75,-52.3,27.675)) ;
#13555=CARTESIAN_POINT('',(70.7,-52.3,27.75)) ;
#13556=CARTESIAN_POINT('',(70.625,-52.3,27.675)) ;
#13557=CARTESIAN_POINT('Origin',(71.75,-52.3,27.75)) ;
#13558=CARTESIAN_POINT('Origin',(71.75,-52.3,27.6)) ;
#13559=CARTESIAN_POINT('',(70.7,-52.3,33.4)) ;
#13560=CARTESIAN_POINT('',(70.7,-52.3,27.6)) ;
#13561=CARTESIAN_POINT('',(70.7183994382024,-52.4957045755694,33.4)) ;
#13562=CARTESIAN_POINT('Origin',(71.75,-52.3,33.4)) ;
#13563=CARTESIAN_POINT('',(70.7183994382024,-52.1042954244305,33.4)) ;
#13564=CARTESIAN_POINT('Ctrl Pts',(70.7183994382024,-52.1042954244305,33.4)) ;
#13565=CARTESIAN_POINT('Ctrl Pts',(70.7319761095756,-52.0327298937054,33.389125081463)) ;
#13566=CARTESIAN_POINT('Ctrl Pts',(70.7531407522363,-51.9623628140592,33.3724123738805)) ;
#13567=CARTESIAN_POINT('Ctrl Pts',(70.8341056071048,-51.7683372704285,33.3125298347947)) ;
#13568=CARTESIAN_POINT('Ctrl Pts',(70.9124422905779,-51.6541937311051,33.2592888082397)) ;
#13569=CARTESIAN_POINT('Ctrl Pts',(71.0924279408069,-51.471154750974,33.1588871128703)) ;
#13570=CARTESIAN_POINT('Ctrl Pts',(71.2082663884949,-51.3895541465464,33.1040987390693)) ;
#13571=CARTESIAN_POINT('Ctrl Pts',(71.4676871756213,-51.2788797863704,33.0155789759107)) ;
#13572=CARTESIAN_POINT('Ctrl Pts',(71.611512060708,-51.25,32.98231678229)) ;
#13573=CARTESIAN_POINT('Ctrl Pts',(71.8811502184983,-51.25,32.9491868010911)) ;
#13574=CARTESIAN_POINT('Ctrl Pts',(72.021484418179,-51.2761809534928,32.9460485518659)) ;
#13575=CARTESIAN_POINT('Ctrl Pts',(72.2790771456966,-51.3824017337057,32.9649830273315)) ;
#13576=CARTESIAN_POINT('Ctrl Pts',(72.3964053699774,-51.4623817460982,32.9864379744825)) ;
#13577=CARTESIAN_POINT('Ctrl Pts',(72.5827722667432,-51.6469682659635,33.0322038118174)) ;
#13578=CARTESIAN_POINT('Ctrl Pts',(72.6641459041156,-51.764644630955,33.0596974322278)) ;
#13579=CARTESIAN_POINT('Ctrl Pts',(72.7727880560022,-52.0240065943841,33.1003519438363)) ;
#13580=CARTESIAN_POINT('Ctrl Pts',(72.8,-52.1658672190012,33.1125413911823)) ;
#13581=CARTESIAN_POINT('Ctrl Pts',(72.8,-52.3,33.1125413911823)) ;
#13582=CARTESIAN_POINT('Ctrl Pts',(72.8,-52.4341327809988,33.1125413911823)) ;
#13583=CARTESIAN_POINT('Ctrl Pts',(72.7727880560022,-52.5759934056159,33.1003519438363)) ;
#13584=CARTESIAN_POINT('Ctrl Pts',(72.6641459041156,-52.835355369045,33.0596974322278)) ;
#13585=CARTESIAN_POINT('Ctrl Pts',(72.5827722667432,-52.9530317340365,33.0322038118174)) ;
#13586=CARTESIAN_POINT('Ctrl Pts',(72.3964053699774,-53.1376182539018,32.9864379744825)) ;
#13587=CARTESIAN_POINT('Ctrl Pts',(72.2790771456966,-53.2175982662943,32.9649830273315)) ;
#13588=CARTESIAN_POINT('Ctrl Pts',(72.021484418179,-53.3238190465072,32.9460485518659)) ;
#13589=CARTESIAN_POINT('Ctrl Pts',(71.8811502184983,-53.35,32.9491868010911)) ;
#13590=CARTESIAN_POINT('Ctrl Pts',(71.611512060708,-53.35,32.98231678229)) ;
#13591=CARTESIAN_POINT('Ctrl Pts',(71.4676871756213,-53.3211202136296,33.0155789759107)) ;
#13592=CARTESIAN_POINT('Ctrl Pts',(71.2082663884949,-53.2104458534536,33.1040987390693)) ;
#13593=CARTESIAN_POINT('Ctrl Pts',(71.0924279408069,-53.128845249026,33.1588871128703)) ;
#13594=CARTESIAN_POINT('Ctrl Pts',(70.9124422905779,-52.9458062688949,33.2592888082397)) ;
#13595=CARTESIAN_POINT('Ctrl Pts',(70.8341056071048,-52.8316627295715,33.3125298347947)) ;
#13596=CARTESIAN_POINT('Ctrl Pts',(70.7531407522362,-52.6376371859408,33.3724123738805)) ;
#13597=CARTESIAN_POINT('Ctrl Pts',(70.7319761095756,-52.5672701062946,33.389125081463)) ;
#13598=CARTESIAN_POINT('Ctrl Pts',(70.7183994382024,-52.4957045755694,33.4)) ;
#13599=CARTESIAN_POINT('Origin',(71.75,-52.3,33.4)) ;
#13600=CARTESIAN_POINT('Origin',(-71.75,52.3,27.675)) ;
#13601=CARTESIAN_POINT('',(-72.8,52.3,27.75)) ;
#13602=CARTESIAN_POINT('',(-72.875,52.3,27.675)) ;
#13603=CARTESIAN_POINT('Origin',(-71.75,52.3,27.75)) ;
#13604=CARTESIAN_POINT('Origin',(-71.75,52.3,27.6)) ;
#13605=CARTESIAN_POINT('',(-72.8,52.3,33.4)) ;
#13606=CARTESIAN_POINT('',(-72.8,52.3,27.6)) ;
#13607=CARTESIAN_POINT('Origin',(-71.75,52.3,33.4)) ;
#13608=CARTESIAN_POINT('Origin',(-71.75,-52.3,27.675)) ;
#13609=CARTESIAN_POINT('',(-72.8,-52.3,27.75)) ;
#13610=CARTESIAN_POINT('',(-72.875,-52.3,27.675)) ;
#13611=CARTESIAN_POINT('Origin',(-71.75,-52.3,27.75)) ;
#13612=CARTESIAN_POINT('Origin',(-71.75,-52.3,27.6)) ;
#13613=CARTESIAN_POINT('',(-72.8,-52.3,33.4)) ;
#13614=CARTESIAN_POINT('',(-72.8,-52.3,27.6)) ;
#13615=CARTESIAN_POINT('Origin',(-71.75,-52.3,33.4)) ;
#13616=CARTESIAN_POINT('Origin',(-84.75,-52.3,33.4)) ;
#13617=CARTESIAN_POINT('',(-84.75,-52.3,34.0309036499789)) ;
#13618=CARTESIAN_POINT('',(-85.8,-52.3,33.4)) ;
#13619=CARTESIAN_POINT('Origin',(-71.75,-52.3,33.4)) ;
#13620=CARTESIAN_POINT('',(-71.75,-52.3,34.0309036499789)) ;
#13621=CARTESIAN_POINT('',(-72.8,-52.3,33.4)) ;
#13622=CARTESIAN_POINT('Origin',(-84.75,52.3,33.4)) ;
#13623=CARTESIAN_POINT('',(-84.75,52.3,34.0309036499789)) ;
#13624=CARTESIAN_POINT('',(-85.8,52.3,33.4)) ;
#13625=CARTESIAN_POINT('Origin',(-71.75,52.3,33.4)) ;
#13626=CARTESIAN_POINT('',(-71.75,52.3,34.0309036499789)) ;
#13627=CARTESIAN_POINT('',(-72.8,52.3,33.4)) ;
#13628=CARTESIAN_POINT('Origin',(71.75,-52.3,33.4)) ;
#13629=CARTESIAN_POINT('Ctrl Pts',(70.7183994382024,-52.4957045755694,33.4)) ;
#13630=CARTESIAN_POINT('Ctrl Pts',(70.7130431211426,-52.4291601614903,33.4042904118456)) ;
#13631=CARTESIAN_POINT('Ctrl Pts',(70.7105358550768,-52.3635187345962,33.4063305804034)) ;
#13632=CARTESIAN_POINT('Ctrl Pts',(70.7105358550768,-52.3,33.4063305804034)) ;
#13633=CARTESIAN_POINT('Ctrl Pts',(70.7105358550768,-52.2364812654038,33.4063305804034)) ;
#13634=CARTESIAN_POINT('Ctrl Pts',(70.7130431211426,-52.1708398385097,33.4042904118456)) ;
#13635=CARTESIAN_POINT('Ctrl Pts',(70.7183994382024,-52.1042954244305,33.4)) ;
#13636=CARTESIAN_POINT('Origin',(72.,-56.3,35.)) ;
#13637=CARTESIAN_POINT('',(69.95,-55.3,35.)) ;
#13638=CARTESIAN_POINT('Origin',(72.,-55.3,35.)) ;
#13639=CARTESIAN_POINT('',(69.95,-49.3,35.)) ;
#13640=CARTESIAN_POINT('',(69.95,-56.3,35.)) ;
#13641=CARTESIAN_POINT('Origin',(72.,-49.3,35.)) ;
#13642=CARTESIAN_POINT('Origin',(84.75,-52.3,33.4)) ;
#13643=CARTESIAN_POINT('',(84.75,-52.3,34.0309036499789)) ;
#13644=CARTESIAN_POINT('',(83.7,-52.3,33.4)) ;
#13645=CARTESIAN_POINT('Origin',(71.75,52.3,33.4)) ;
#13646=CARTESIAN_POINT('Ctrl Pts',(70.7183994382024,52.1042954244305,33.4)) ;
#13647=CARTESIAN_POINT('Ctrl Pts',(70.7130431211426,52.1708398385097,33.4042904118456)) ;
#13648=CARTESIAN_POINT('Ctrl Pts',(70.7105358550768,52.2364812654038,33.4063305804034)) ;
#13649=CARTESIAN_POINT('Ctrl Pts',(70.7105358550768,52.3,33.4063305804034)) ;
#13650=CARTESIAN_POINT('Ctrl Pts',(70.7105358550768,52.3635187345962,33.4063305804034)) ;
#13651=CARTESIAN_POINT('Ctrl Pts',(70.7130431211426,52.4291601614903,33.4042904118456)) ;
#13652=CARTESIAN_POINT('Ctrl Pts',(70.7183994382024,52.4957045755694,33.4)) ;
#13653=CARTESIAN_POINT('Origin',(72.,-56.3,35.)) ;
#13654=CARTESIAN_POINT('',(69.95,49.3,35.)) ;
#13655=CARTESIAN_POINT('Origin',(72.,49.3,35.)) ;
#13656=CARTESIAN_POINT('',(69.95,55.3,35.)) ;
#13657=CARTESIAN_POINT('',(69.95,-56.3,35.)) ;
#13658=CARTESIAN_POINT('Origin',(72.,55.3,35.)) ;
#13659=CARTESIAN_POINT('Origin',(84.75,52.3,33.4)) ;
#13660=CARTESIAN_POINT('',(84.75,52.3,34.0309036499789)) ;
#13661=CARTESIAN_POINT('',(83.7,52.3,33.4)) ;
#13662=CARTESIAN_POINT('Origin',(88.75,-45.,50.)) ;
#13663=CARTESIAN_POINT('',(88.0811225508981,-46.15,50.)) ;
#13664=CARTESIAN_POINT('',(88.25,-45.,51.15)) ;
#13665=CARTESIAN_POINT('Ctrl Pts',(88.0811225508981,-46.15,50.)) ;
#13666=CARTESIAN_POINT('Ctrl Pts',(88.0811225508981,-46.15,50.1453034266508)) ;
#13667=CARTESIAN_POINT('Ctrl Pts',(88.0902531665979,-46.1207924457676,50.2996897552291)) ;
#13668=CARTESIAN_POINT('Ctrl Pts',(88.1226395702438,-46.0031862805799,50.5827581865916)) ;
#13669=CARTESIAN_POINT('Ctrl Pts',(88.1453650465612,-45.9148280935687,50.7115175031603)) ;
#13670=CARTESIAN_POINT('Ctrl Pts',(88.1875729412465,-45.7115428603744,50.9148027363547)) ;
#13671=CARTESIAN_POINT('Ctrl Pts',(88.2098812441699,-45.5827731705935,51.0031805967208)) ;
#13672=CARTESIAN_POINT('Ctrl Pts',(88.2413009851215,-45.2996672843957,51.1208012401597)) ;
#13673=CARTESIAN_POINT('Ctrl Pts',(88.25,-45.1452671817106,51.15)) ;
#13674=CARTESIAN_POINT('Ctrl Pts',(88.25,-45.,51.15)) ;
#13675=CARTESIAN_POINT('Ctrl Pts',(88.25,-45.,51.15)) ;
#13676=CARTESIAN_POINT('Ctrl Pts',(88.25,-44.8547328182893,51.15)) ;
#13677=CARTESIAN_POINT('Ctrl Pts',(88.2413009851215,-44.7003327156043,51.1208012401597)) ;
#13678=CARTESIAN_POINT('Ctrl Pts',(88.2098812441699,-44.4172268294065,51.0031805967208)) ;
#13679=CARTESIAN_POINT('Ctrl Pts',(88.1875729412465,-44.2884571396256,50.9148027363547)) ;
#13680=CARTESIAN_POINT('Ctrl Pts',(88.1453650465612,-44.0851719064313,50.7115175031603)) ;
#13681=CARTESIAN_POINT('Ctrl Pts',(88.1226395702438,-43.9968137194201,50.5827581865916)) ;
#13682=CARTESIAN_POINT('Ctrl Pts',(88.0902531665979,-43.8792075542324,50.2996897552291)) ;
#13683=CARTESIAN_POINT('Ctrl Pts',(88.0811225508981,-43.85,50.1453034266508)) ;
#13684=CARTESIAN_POINT('Ctrl Pts',(88.0811225508981,-43.85,49.8546965733492)) ;
#13685=CARTESIAN_POINT('Ctrl Pts',(88.0902531665979,-43.8792075542324,49.7003102447709)) ;
#13686=CARTESIAN_POINT('Ctrl Pts',(88.1226395702438,-43.9968137194201,49.4172418134084)) ;
#13687=CARTESIAN_POINT('Ctrl Pts',(88.1453650465612,-44.0851719064313,49.2884824968397)) ;
#13688=CARTESIAN_POINT('Ctrl Pts',(88.1875729412465,-44.2884571396256,49.0851972636453)) ;
#13689=CARTESIAN_POINT('Ctrl Pts',(88.2098812441699,-44.4172268294065,48.9968194032792)) ;
#13690=CARTESIAN_POINT('Ctrl Pts',(88.2413009851215,-44.7003327156043,48.8791987598403)) ;
#13691=CARTESIAN_POINT('Ctrl Pts',(88.25,-44.8547328182894,48.85)) ;
#13692=CARTESIAN_POINT('Ctrl Pts',(88.25,-45.1452671817106,48.85)) ;
#13693=CARTESIAN_POINT('Ctrl Pts',(88.2413009851215,-45.2996672843957,48.8791987598403)) ;
#13694=CARTESIAN_POINT('Ctrl Pts',(88.2098812441699,-45.5827731705935,48.9968194032792)) ;
#13695=CARTESIAN_POINT('Ctrl Pts',(88.1875729412465,-45.7115428603744,49.0851972636453)) ;
#13696=CARTESIAN_POINT('Ctrl Pts',(88.1453650465612,-45.9148280935687,49.2884824968397)) ;
#13697=CARTESIAN_POINT('Ctrl Pts',(88.1226395702438,-46.0031862805799,49.4172418134084)) ;
#13698=CARTESIAN_POINT('Ctrl Pts',(88.0902531665979,-46.1207924457676,49.7003102447709)) ;
#13699=CARTESIAN_POINT('Ctrl Pts',(88.0811225508981,-46.15,49.8546965733492)) ;
#13700=CARTESIAN_POINT('Ctrl Pts',(88.0811225508981,-46.15,50.)) ;
#13701=CARTESIAN_POINT('',(87.2,-45.,51.15)) ;
#13702=CARTESIAN_POINT('',(88.75,-45.,51.15)) ;
#13703=CARTESIAN_POINT('',(86.9666155414412,-43.85,50.)) ;
#13704=CARTESIAN_POINT('Ctrl Pts',(86.9666155414412,-43.85,50.)) ;
#13705=CARTESIAN_POINT('Ctrl Pts',(86.9666155414412,-43.85,50.1461583267558)) ;
#13706=CARTESIAN_POINT('Ctrl Pts',(86.9796573686722,-43.8795285636834,50.3008398252782)) ;
#13707=CARTESIAN_POINT('Ctrl Pts',(87.0250928731078,-43.9973311263918,50.5836234155483)) ;
#13708=CARTESIAN_POINT('Ctrl Pts',(87.0566642086003,-44.0855389722715,50.7118845690005)) ;
#13709=CARTESIAN_POINT('Ctrl Pts',(87.1147290825117,-44.2880237720613,50.9143693687904)) ;
#13710=CARTESIAN_POINT('Ctrl Pts',(87.1452181894816,-44.4163199277569,51.0026469087132)) ;
#13711=CARTESIAN_POINT('Ctrl Pts',(87.188113941166,-44.6992388624653,51.1205025788281)) ;
#13712=CARTESIAN_POINT('Ctrl Pts',(87.2,-44.8539739365597,51.15)) ;
#13713=CARTESIAN_POINT('Ctrl Pts',(87.2,-45.,51.15)) ;
#13714=CARTESIAN_POINT('Ctrl Pts',(87.2,-45.,51.15)) ;
#13715=CARTESIAN_POINT('Ctrl Pts',(87.2,-45.1460260634403,51.15)) ;
#13716=CARTESIAN_POINT('Ctrl Pts',(87.188113941166,-45.3007611375347,51.1205025788281)) ;
#13717=CARTESIAN_POINT('Ctrl Pts',(87.1452181894816,-45.5836800722431,51.0026469087132)) ;
#13718=CARTESIAN_POINT('Ctrl Pts',(87.1147290825117,-45.7119762279387,50.9143693687904)) ;
#13719=CARTESIAN_POINT('Ctrl Pts',(87.0566642086003,-45.9144610277285,50.7118845690005)) ;
#13720=CARTESIAN_POINT('Ctrl Pts',(87.0250928731078,-46.0026688736082,50.5836234155483)) ;
#13721=CARTESIAN_POINT('Ctrl Pts',(86.9796573686722,-46.1204714363166,50.3008398252782)) ;
#13722=CARTESIAN_POINT('Ctrl Pts',(86.9666155414412,-46.15,50.1461583267558)) ;
#13723=CARTESIAN_POINT('Ctrl Pts',(86.9666155414412,-46.15,49.8538416732442)) ;
#13724=CARTESIAN_POINT('Ctrl Pts',(86.9796573686722,-46.1204714363166,49.6991601747218)) ;
#13725=CARTESIAN_POINT('Ctrl Pts',(87.0250928731078,-46.0026688736082,49.4163765844517)) ;
#13726=CARTESIAN_POINT('Ctrl Pts',(87.0566642086003,-45.9144610277285,49.2881154309995)) ;
#13727=CARTESIAN_POINT('Ctrl Pts',(87.1147290825117,-45.7119762279387,49.0856306312096)) ;
#13728=CARTESIAN_POINT('Ctrl Pts',(87.1452181894816,-45.5836800722431,48.9973530912868)) ;
#13729=CARTESIAN_POINT('Ctrl Pts',(87.188113941166,-45.3007611375347,48.8794974211719)) ;
#13730=CARTESIAN_POINT('Ctrl Pts',(87.2,-45.1460260634403,48.85)) ;
#13731=CARTESIAN_POINT('Ctrl Pts',(87.2,-44.8539739365597,48.85)) ;
#13732=CARTESIAN_POINT('Ctrl Pts',(87.188113941166,-44.6992388624653,48.8794974211719)) ;
#13733=CARTESIAN_POINT('Ctrl Pts',(87.1452181894816,-44.4163199277569,48.9973530912868)) ;
#13734=CARTESIAN_POINT('Ctrl Pts',(87.1147290825117,-44.2880237720613,49.0856306312096)) ;
#13735=CARTESIAN_POINT('Ctrl Pts',(87.0566642086003,-44.0855389722715,49.2881154309995)) ;
#13736=CARTESIAN_POINT('Ctrl Pts',(87.0250928731078,-43.9973311263918,49.4163765844517)) ;
#13737=CARTESIAN_POINT('Ctrl Pts',(86.9796573686722,-43.8795285636834,49.6991601747218)) ;
#13738=CARTESIAN_POINT('Ctrl Pts',(86.9666155414412,-43.85,49.8538416732443)) ;
#13739=CARTESIAN_POINT('Ctrl Pts',(86.9666155414412,-43.85,50.)) ;
#13740=CARTESIAN_POINT('Origin',(84.25,-45.,55.)) ;
#13741=CARTESIAN_POINT('',(81.3,-45.,55.)) ;
#13742=CARTESIAN_POINT('Origin',(84.25,-45.,55.)) ;
#13743=CARTESIAN_POINT('',(81.3,-45.,41.)) ;
#13744=CARTESIAN_POINT('',(81.3,-45.,55.)) ;
#13745=CARTESIAN_POINT('Origin',(84.25,-45.,41.)) ;
#13746=CARTESIAN_POINT('Origin',(84.25,-45.,41.)) ;
#13747=CARTESIAN_POINT('Origin',(88.75,45.,50.)) ;
#13748=CARTESIAN_POINT('',(88.0811225508981,43.85,50.)) ;
#13749=CARTESIAN_POINT('',(88.25,45.,51.15)) ;
#13750=CARTESIAN_POINT('Ctrl Pts',(88.0811225508981,43.85,50.)) ;
#13751=CARTESIAN_POINT('Ctrl Pts',(88.0811225508981,43.85,50.1453034266508)) ;
#13752=CARTESIAN_POINT('Ctrl Pts',(88.0902531665979,43.8792075542324,50.2996897552291)) ;
#13753=CARTESIAN_POINT('Ctrl Pts',(88.1226395702438,43.9968137194201,50.5827581865916)) ;
#13754=CARTESIAN_POINT('Ctrl Pts',(88.1453650465612,44.0851719064313,50.7115175031603)) ;
#13755=CARTESIAN_POINT('Ctrl Pts',(88.1875729412465,44.2884571396256,50.9148027363547)) ;
#13756=CARTESIAN_POINT('Ctrl Pts',(88.2098812441699,44.4172268294065,51.0031805967208)) ;
#13757=CARTESIAN_POINT('Ctrl Pts',(88.2413009851215,44.7003327156042,51.1208012401597)) ;
#13758=CARTESIAN_POINT('Ctrl Pts',(88.25,44.8547328182894,51.15)) ;
#13759=CARTESIAN_POINT('Ctrl Pts',(88.25,45.,51.15)) ;
#13760=CARTESIAN_POINT('Ctrl Pts',(88.25,45.,51.15)) ;
#13761=CARTESIAN_POINT('Ctrl Pts',(88.25,45.1452671817106,51.15)) ;
#13762=CARTESIAN_POINT('Ctrl Pts',(88.2413009851215,45.2996672843957,51.1208012401597)) ;
#13763=CARTESIAN_POINT('Ctrl Pts',(88.2098812441699,45.5827731705935,51.0031805967208)) ;
#13764=CARTESIAN_POINT('Ctrl Pts',(88.1875729412465,45.7115428603744,50.9148027363547)) ;
#13765=CARTESIAN_POINT('Ctrl Pts',(88.1453650465612,45.9148280935687,50.7115175031603)) ;
#13766=CARTESIAN_POINT('Ctrl Pts',(88.1226395702438,46.0031862805799,50.5827581865916)) ;
#13767=CARTESIAN_POINT('Ctrl Pts',(88.0902531665979,46.1207924457676,50.2996897552291)) ;
#13768=CARTESIAN_POINT('Ctrl Pts',(88.0811225508981,46.15,50.1453034266508)) ;
#13769=CARTESIAN_POINT('Ctrl Pts',(88.0811225508981,46.15,49.8546965733492)) ;
#13770=CARTESIAN_POINT('Ctrl Pts',(88.0902531665979,46.1207924457676,49.7003102447709)) ;
#13771=CARTESIAN_POINT('Ctrl Pts',(88.1226395702438,46.0031862805799,49.4172418134084)) ;
#13772=CARTESIAN_POINT('Ctrl Pts',(88.1453650465612,45.9148280935687,49.2884824968397)) ;
#13773=CARTESIAN_POINT('Ctrl Pts',(88.1875729412465,45.7115428603744,49.0851972636453)) ;
#13774=CARTESIAN_POINT('Ctrl Pts',(88.2098812441699,45.5827731705935,48.9968194032792)) ;
#13775=CARTESIAN_POINT('Ctrl Pts',(88.2413009851215,45.2996672843957,48.8791987598403)) ;
#13776=CARTESIAN_POINT('Ctrl Pts',(88.25,45.1452671817106,48.85)) ;
#13777=CARTESIAN_POINT('Ctrl Pts',(88.25,44.8547328182894,48.85)) ;
#13778=CARTESIAN_POINT('Ctrl Pts',(88.2413009851215,44.7003327156043,48.8791987598403)) ;
#13779=CARTESIAN_POINT('Ctrl Pts',(88.2098812441699,44.4172268294065,48.9968194032792)) ;
#13780=CARTESIAN_POINT('Ctrl Pts',(88.1875729412465,44.2884571396256,49.0851972636453)) ;
#13781=CARTESIAN_POINT('Ctrl Pts',(88.1453650465612,44.0851719064313,49.2884824968397)) ;
#13782=CARTESIAN_POINT('Ctrl Pts',(88.1226395702438,43.9968137194201,49.4172418134084)) ;
#13783=CARTESIAN_POINT('Ctrl Pts',(88.0902531665979,43.8792075542324,49.7003102447709)) ;
#13784=CARTESIAN_POINT('Ctrl Pts',(88.0811225508981,43.85,49.8546965733492)) ;
#13785=CARTESIAN_POINT('Ctrl Pts',(88.0811225508981,43.85,50.)) ;
#13786=CARTESIAN_POINT('',(87.2,45.,51.15)) ;
#13787=CARTESIAN_POINT('',(88.75,45.,51.15)) ;
#13788=CARTESIAN_POINT('',(86.9666155414412,46.15,50.)) ;
#13789=CARTESIAN_POINT('Ctrl Pts',(86.9666155414412,46.15,50.)) ;
#13790=CARTESIAN_POINT('Ctrl Pts',(86.9666155414412,46.15,50.1461583267558)) ;
#13791=CARTESIAN_POINT('Ctrl Pts',(86.9796573686722,46.1204714363166,50.3008398252782)) ;
#13792=CARTESIAN_POINT('Ctrl Pts',(87.0250928731078,46.0026688736082,50.5836234155483)) ;
#13793=CARTESIAN_POINT('Ctrl Pts',(87.0566642086003,45.9144610277285,50.7118845690005)) ;
#13794=CARTESIAN_POINT('Ctrl Pts',(87.1147290825117,45.7119762279387,50.9143693687904)) ;
#13795=CARTESIAN_POINT('Ctrl Pts',(87.1452181894816,45.5836800722431,51.0026469087132)) ;
#13796=CARTESIAN_POINT('Ctrl Pts',(87.188113941166,45.3007611375347,51.1205025788281)) ;
#13797=CARTESIAN_POINT('Ctrl Pts',(87.2,45.1460260634403,51.15)) ;
#13798=CARTESIAN_POINT('Ctrl Pts',(87.2,45.,51.15)) ;
#13799=CARTESIAN_POINT('Ctrl Pts',(87.2,45.,51.15)) ;
#13800=CARTESIAN_POINT('Ctrl Pts',(87.2,44.8539739365597,51.15)) ;
#13801=CARTESIAN_POINT('Ctrl Pts',(87.188113941166,44.6992388624653,51.1205025788281)) ;
#13802=CARTESIAN_POINT('Ctrl Pts',(87.1452181894816,44.4163199277569,51.0026469087132)) ;
#13803=CARTESIAN_POINT('Ctrl Pts',(87.1147290825117,44.2880237720613,50.9143693687904)) ;
#13804=CARTESIAN_POINT('Ctrl Pts',(87.0566642086003,44.0855389722715,50.7118845690005)) ;
#13805=CARTESIAN_POINT('Ctrl Pts',(87.0250928731078,43.9973311263918,50.5836234155483)) ;
#13806=CARTESIAN_POINT('Ctrl Pts',(86.9796573686722,43.8795285636834,50.3008398252782)) ;
#13807=CARTESIAN_POINT('Ctrl Pts',(86.9666155414412,43.85,50.1461583267558)) ;
#13808=CARTESIAN_POINT('Ctrl Pts',(86.9666155414412,43.85,49.8538416732442)) ;
#13809=CARTESIAN_POINT('Ctrl Pts',(86.9796573686722,43.8795285636834,49.6991601747218)) ;
#13810=CARTESIAN_POINT('Ctrl Pts',(87.0250928731078,43.9973311263918,49.4163765844517)) ;
#13811=CARTESIAN_POINT('Ctrl Pts',(87.0566642086003,44.0855389722715,49.2881154309995)) ;
#13812=CARTESIAN_POINT('Ctrl Pts',(87.1147290825117,44.2880237720613,49.0856306312096)) ;
#13813=CARTESIAN_POINT('Ctrl Pts',(87.1452181894816,44.4163199277569,48.9973530912868)) ;
#13814=CARTESIAN_POINT('Ctrl Pts',(87.188113941166,44.6992388624653,48.8794974211719)) ;
#13815=CARTESIAN_POINT('Ctrl Pts',(87.2,44.8539739365597,48.85)) ;
#13816=CARTESIAN_POINT('Ctrl Pts',(87.2,45.1460260634403,48.85)) ;
#13817=CARTESIAN_POINT('Ctrl Pts',(87.188113941166,45.3007611375347,48.8794974211719)) ;
#13818=CARTESIAN_POINT('Ctrl Pts',(87.1452181894816,45.5836800722431,48.9973530912868)) ;
#13819=CARTESIAN_POINT('Ctrl Pts',(87.1147290825117,45.7119762279387,49.0856306312096)) ;
#13820=CARTESIAN_POINT('Ctrl Pts',(87.0566642086003,45.9144610277285,49.2881154309995)) ;
#13821=CARTESIAN_POINT('Ctrl Pts',(87.0250928731078,46.0026688736082,49.4163765844517)) ;
#13822=CARTESIAN_POINT('Ctrl Pts',(86.9796573686722,46.1204714363166,49.6991601747218)) ;
#13823=CARTESIAN_POINT('Ctrl Pts',(86.9666155414412,46.15,49.8538416732442)) ;
#13824=CARTESIAN_POINT('Ctrl Pts',(86.9666155414412,46.15,50.)) ;
#13825=CARTESIAN_POINT('Origin',(84.25,45.,55.)) ;
#13826=CARTESIAN_POINT('',(81.3,45.,55.)) ;
#13827=CARTESIAN_POINT('Origin',(84.25,45.,55.)) ;
#13828=CARTESIAN_POINT('',(81.3,45.,41.)) ;
#13829=CARTESIAN_POINT('',(81.3,45.,55.)) ;
#13830=CARTESIAN_POINT('Origin',(84.25,45.,41.)) ;
#13831=CARTESIAN_POINT('Origin',(84.25,45.,41.)) ;
#13832=CARTESIAN_POINT('Origin',(77.,-4.,35.)) ;
#13833=CARTESIAN_POINT('',(74.95,2.3,35.)) ;
#13834=CARTESIAN_POINT('Origin',(77.,2.3,35.)) ;
#13835=CARTESIAN_POINT('',(74.95,3.3,35.)) ;
#13836=CARTESIAN_POINT('',(74.95,-4.,35.)) ;
#13837=CARTESIAN_POINT('Origin',(77.,3.3,35.)) ;
#13838=CARTESIAN_POINT('Origin',(77.,-4.,35.)) ;
#13839=CARTESIAN_POINT('',(74.95,-3.3,35.)) ;
#13840=CARTESIAN_POINT('Origin',(77.,-3.3,35.)) ;
#13841=CARTESIAN_POINT('',(74.95,-2.3,35.)) ;
#13842=CARTESIAN_POINT('',(74.95,-4.,35.)) ;
#13843=CARTESIAN_POINT('Origin',(77.,-2.3,35.)) ;
#13844=CARTESIAN_POINT('Origin',(72.,-56.3,35.)) ;
#13845=CARTESIAN_POINT('',(73.69525,3.3,36.1526610245428)) ;
#13846=CARTESIAN_POINT('',(73.69525,2.3,36.1526610245428)) ;
#13847=CARTESIAN_POINT('',(73.69525,-56.3,36.1526610245428)) ;
#13848=CARTESIAN_POINT('',(73.5,3.3,33.6026811387518)) ;
#13849=CARTESIAN_POINT('Origin',(72.,3.3,35.)) ;
#13850=CARTESIAN_POINT('',(73.5,2.3,33.6026811387518)) ;
#13851=CARTESIAN_POINT('',(73.5,-56.3,33.6026811387518)) ;
#13852=CARTESIAN_POINT('Origin',(72.,2.3,35.)) ;
#13853=CARTESIAN_POINT('Origin',(72.,-56.3,35.)) ;
#13854=CARTESIAN_POINT('',(73.69525,-2.3,36.1526610245428)) ;
#13855=CARTESIAN_POINT('',(73.69525,-3.3,36.1526610245428)) ;
#13856=CARTESIAN_POINT('',(73.69525,-56.3,36.1526610245428)) ;
#13857=CARTESIAN_POINT('',(73.5,-2.3,33.6026811387518)) ;
#13858=CARTESIAN_POINT('Origin',(72.,-2.3,35.)) ;
#13859=CARTESIAN_POINT('',(73.5,-3.3,33.6026811387518)) ;
#13860=CARTESIAN_POINT('',(73.5,-56.3,33.6026811387518)) ;
#13861=CARTESIAN_POINT('Origin',(72.,-3.3,35.)) ;
#13862=CARTESIAN_POINT('Origin',(73.5,-3.3,30.)) ;
#13863=CARTESIAN_POINT('',(73.5,-2.3,30.)) ;
#13864=CARTESIAN_POINT('',(73.5,-2.3,30.)) ;
#13865=CARTESIAN_POINT('',(73.5,-3.3,30.)) ;
#13866=CARTESIAN_POINT('',(73.5,-3.3,30.)) ;
#13867=CARTESIAN_POINT('',(73.5,-3.3,30.)) ;
#13868=CARTESIAN_POINT('Origin',(77.375,-2.3,34.25)) ;
#13869=CARTESIAN_POINT('',(80.5,-2.3,35.)) ;
#13870=CARTESIAN_POINT('Origin',(77.,-2.3,35.)) ;
#13871=CARTESIAN_POINT('',(81.25,-2.3,35.)) ;
#13872=CARTESIAN_POINT('',(80.5,-2.3,35.)) ;
#13873=CARTESIAN_POINT('',(81.25,-2.3,30.)) ;
#13874=CARTESIAN_POINT('',(81.25,-2.3,31.675)) ;
#13875=CARTESIAN_POINT('',(81.25,-2.3,30.)) ;
#13876=CARTESIAN_POINT('Origin',(73.5,2.3,30.)) ;
#13877=CARTESIAN_POINT('',(73.5,3.3,30.)) ;
#13878=CARTESIAN_POINT('',(73.5,3.3,30.)) ;
#13879=CARTESIAN_POINT('',(73.5,2.3,30.)) ;
#13880=CARTESIAN_POINT('',(73.5,2.3,30.)) ;
#13881=CARTESIAN_POINT('',(73.5,2.3,30.)) ;
#13882=CARTESIAN_POINT('Origin',(77.375,3.3,34.25)) ;
#13883=CARTESIAN_POINT('',(80.5,3.3,35.)) ;
#13884=CARTESIAN_POINT('Origin',(77.,3.3,35.)) ;
#13885=CARTESIAN_POINT('',(81.25,3.3,35.)) ;
#13886=CARTESIAN_POINT('',(80.5,3.3,35.)) ;
#13887=CARTESIAN_POINT('',(81.25,3.3,30.)) ;
#13888=CARTESIAN_POINT('',(81.25,3.3,31.675)) ;
#13889=CARTESIAN_POINT('',(81.25,3.3,30.)) ;
#13890=CARTESIAN_POINT('Origin',(43.625,55.05,38.85)) ;
#13891=CARTESIAN_POINT('',(-87.25,55.3,38.6)) ;
#13892=CARTESIAN_POINT('',(-87.25,54.8,39.1)) ;
#13893=CARTESIAN_POINT('',(-87.25,57.55,36.35)) ;
#13894=CARTESIAN_POINT('',(87.25,54.8,39.1)) ;
#13895=CARTESIAN_POINT('',(43.625,54.8,39.1)) ;
#13896=CARTESIAN_POINT('',(87.25,55.3,38.6)) ;
#13897=CARTESIAN_POINT('',(87.25,56.05,37.85)) ;
#13898=CARTESIAN_POINT('',(43.625,55.3,38.6)) ;
#13899=CARTESIAN_POINT('Origin',(87.25,55.3,29.1)) ;
#13900=CARTESIAN_POINT('',(87.25,55.3,29.1)) ;
#13901=CARTESIAN_POINT('',(87.25,55.3,29.1)) ;
#13902=CARTESIAN_POINT('',(69.25,55.3,29.1)) ;
#13903=CARTESIAN_POINT('',(87.25,55.3,29.1)) ;
#13904=CARTESIAN_POINT('',(-69.25,55.3,29.1)) ;
#13905=CARTESIAN_POINT('',(87.25,55.3,29.1)) ;
#13906=CARTESIAN_POINT('',(-87.25,55.3,29.1)) ;
#13907=CARTESIAN_POINT('',(87.25,55.3,29.1)) ;
#13908=CARTESIAN_POINT('',(-87.25,55.3,29.1)) ;
#13909=CARTESIAN_POINT('Origin',(87.25,49.3,29.1)) ;
#13910=CARTESIAN_POINT('',(87.25,47.6457513110646,39.1)) ;
#13911=CARTESIAN_POINT('',(87.25,-55.3,39.1)) ;
#13912=CARTESIAN_POINT('',(87.25,47.6457513110646,38.6)) ;
#13913=CARTESIAN_POINT('',(87.25,47.6457513110646,46.8)) ;
#13914=CARTESIAN_POINT('',(87.25,42.3542486889354,38.6)) ;
#13915=CARTESIAN_POINT('',(87.25,47.15,38.6)) ;
#13916=CARTESIAN_POINT('',(87.25,42.3542486889354,39.1)) ;
#13917=CARTESIAN_POINT('',(87.25,42.3542486889354,46.8)) ;
#13918=CARTESIAN_POINT('',(87.25,-42.3542486889354,39.1)) ;
#13919=CARTESIAN_POINT('',(87.25,-55.3,39.1)) ;
#13920=CARTESIAN_POINT('',(87.25,-42.3542486889354,38.6)) ;
#13921=CARTESIAN_POINT('',(87.25,-42.3542486889354,46.8)) ;
#13922=CARTESIAN_POINT('',(87.25,-47.6457513110646,38.6)) ;
#13923=CARTESIAN_POINT('',(87.25,2.15,38.6)) ;
#13924=CARTESIAN_POINT('',(87.25,-47.6457513110646,39.1)) ;
#13925=CARTESIAN_POINT('',(87.25,-47.6457513110646,46.8)) ;
#13926=CARTESIAN_POINT('',(87.25,-54.8,39.1)) ;
#13927=CARTESIAN_POINT('',(87.25,-55.3,39.1)) ;
#13928=CARTESIAN_POINT('',(87.25,-55.3,38.6)) ;
#13929=CARTESIAN_POINT('',(87.25,-31.4,62.5)) ;
#13930=CARTESIAN_POINT('',(87.25,-55.3,29.1)) ;
#13931=CARTESIAN_POINT('',(87.25,-55.3,29.1)) ;
#13932=CARTESIAN_POINT('',(87.25,-59.3,29.1)) ;
#13933=CARTESIAN_POINT('',(87.25,-59.3,29.1)) ;
#13934=CARTESIAN_POINT('',(87.25,-59.3,27.6)) ;
#13935=CARTESIAN_POINT('',(87.25,-45.3,29.1)) ;
#13936=CARTESIAN_POINT('',(87.25,-45.3,27.6)) ;
#13937=CARTESIAN_POINT('',(87.25,45.3,29.1)) ;
#13938=CARTESIAN_POINT('',(87.25,-55.3,29.1)) ;
#13939=CARTESIAN_POINT('',(87.25,45.3,27.6)) ;
#13940=CARTESIAN_POINT('',(87.25,59.3,29.1)) ;
#13941=CARTESIAN_POINT('',(87.25,59.3,27.6)) ;
#13942=CARTESIAN_POINT('',(87.25,45.3,29.1)) ;
#13943=CARTESIAN_POINT('Origin',(-43.625,-55.05,38.85)) ;
#13944=CARTESIAN_POINT('',(-87.25,-54.8,39.1)) ;
#13945=CARTESIAN_POINT('',(-43.625,-54.8,39.1)) ;
#13946=CARTESIAN_POINT('',(-87.25,-55.3,38.6)) ;
#13947=CARTESIAN_POINT('',(-87.25,-29.9,64.)) ;
#13948=CARTESIAN_POINT('',(-43.625,-55.3,38.6)) ;
#13949=CARTESIAN_POINT('Origin',(-87.25,-55.3,29.1)) ;
#13950=CARTESIAN_POINT('',(-87.25,-55.3,29.1)) ;
#13951=CARTESIAN_POINT('',(-87.25,-55.3,29.1)) ;
#13952=CARTESIAN_POINT('',(-69.25,-55.3,29.1)) ;
#13953=CARTESIAN_POINT('',(-87.25,-55.3,29.1)) ;
#13954=CARTESIAN_POINT('',(69.25,-55.3,29.1)) ;
#13955=CARTESIAN_POINT('',(-87.25,-55.3,29.1)) ;
#13956=CARTESIAN_POINT('',(-87.25,-55.3,29.1)) ;
#13957=CARTESIAN_POINT('Origin',(84.25,-45.,46.8)) ;
#13958=CARTESIAN_POINT('',(80.25,-45.,55.)) ;
#13959=CARTESIAN_POINT('Origin',(84.25,-45.,55.)) ;
#13960=CARTESIAN_POINT('',(80.25,-45.,38.6)) ;
#13961=CARTESIAN_POINT('',(80.25,-45.,46.8)) ;
#13962=CARTESIAN_POINT('',(81.25,-47.6457513110646,38.6)) ;
#13963=CARTESIAN_POINT('Origin',(84.25,-45.,38.6)) ;
#13964=CARTESIAN_POINT('',(81.25,-47.6457513110646,39.1)) ;
#13965=CARTESIAN_POINT('',(81.25,-47.6457513110646,46.8)) ;
#13966=CARTESIAN_POINT('Origin',(84.25,-45.,39.1)) ;
#13967=CARTESIAN_POINT('Origin',(84.25,-45.,38.6)) ;
#13968=CARTESIAN_POINT('',(81.25,-42.3542486889354,39.1)) ;
#13969=CARTESIAN_POINT('Origin',(84.25,-45.,39.1)) ;
#13970=CARTESIAN_POINT('',(81.25,-42.3542486889354,38.6)) ;
#13971=CARTESIAN_POINT('',(81.25,-42.3542486889354,46.8)) ;
#13972=CARTESIAN_POINT('Origin',(84.25,-45.,38.6)) ;
#13973=CARTESIAN_POINT('Origin',(88.25,-45.,38.6)) ;
#13974=CARTESIAN_POINT('Origin',(88.25,-45.,38.6)) ;
#13975=CARTESIAN_POINT('',(81.25,2.15,38.6)) ;
#13976=CARTESIAN_POINT('Origin',(84.25,-45.,55.)) ;
#13977=CARTESIAN_POINT('Origin',(81.25,49.3,29.1)) ;
#13978=CARTESIAN_POINT('',(81.25,42.3542486889354,39.1)) ;
#13979=CARTESIAN_POINT('',(81.25,49.3,39.1)) ;
#13980=CARTESIAN_POINT('',(81.25,42.3542486889354,38.6)) ;
#13981=CARTESIAN_POINT('',(81.25,42.3542486889354,46.8)) ;
#13982=CARTESIAN_POINT('',(81.25,47.6457513110646,38.6)) ;
#13983=CARTESIAN_POINT('',(81.25,47.15,38.6)) ;
#13984=CARTESIAN_POINT('',(81.25,47.6457513110646,39.1)) ;
#13985=CARTESIAN_POINT('',(81.25,47.6457513110646,46.8)) ;
#13986=CARTESIAN_POINT('',(81.25,49.3,39.1)) ;
#13987=CARTESIAN_POINT('',(81.25,49.3,39.1)) ;
#13988=CARTESIAN_POINT('',(81.25,49.3,29.1)) ;
#13989=CARTESIAN_POINT('',(81.25,49.3,29.1)) ;
#13990=CARTESIAN_POINT('',(81.25,45.3,29.1)) ;
#13991=CARTESIAN_POINT('',(81.25,49.3,29.1)) ;
#13992=CARTESIAN_POINT('',(81.25,-45.3,29.1)) ;
#13993=CARTESIAN_POINT('',(81.25,49.3,29.1)) ;
#13994=CARTESIAN_POINT('',(81.25,-49.3,29.1)) ;
#13995=CARTESIAN_POINT('',(81.25,49.3,29.1)) ;
#13996=CARTESIAN_POINT('',(81.25,-49.3,39.1)) ;
#13997=CARTESIAN_POINT('',(81.25,-49.3,29.1)) ;
#13998=CARTESIAN_POINT('',(81.25,49.3,39.1)) ;
#13999=CARTESIAN_POINT('',(81.25,2.3,35.)) ;
#14000=CARTESIAN_POINT('',(81.25,25.8,35.)) ;
#14001=CARTESIAN_POINT('',(81.25,2.3,30.)) ;
#14002=CARTESIAN_POINT('',(81.25,2.3,31.675)) ;
#14003=CARTESIAN_POINT('',(81.25,25.8,30.)) ;
#14004=CARTESIAN_POINT('',(81.25,-3.3,35.)) ;
#14005=CARTESIAN_POINT('',(81.25,23.,35.)) ;
#14006=CARTESIAN_POINT('',(81.25,-3.3,30.)) ;
#14007=CARTESIAN_POINT('',(81.25,-3.3,31.675)) ;
#14008=CARTESIAN_POINT('',(81.25,23.,30.)) ;
#14009=CARTESIAN_POINT('Origin',(0.,52.3,39.1)) ;
#14010=CARTESIAN_POINT('Origin',(84.25,45.,39.1)) ;
#14011=CARTESIAN_POINT('Origin',(81.25,-3.3,30.)) ;
#14012=CARTESIAN_POINT('',(81.25,-3.3,30.)) ;
#14013=CARTESIAN_POINT('Origin',(80.5,-3.3,35.)) ;
#14014=CARTESIAN_POINT('',(80.5,-3.3,35.)) ;
#14015=CARTESIAN_POINT('',(80.5,-3.3,35.)) ;
#14016=CARTESIAN_POINT('',(80.5,-3.3,35.)) ;
#14017=CARTESIAN_POINT('Origin',(77.,-3.3,35.)) ;
#14018=CARTESIAN_POINT('Origin',(77.,-3.3,35.)) ;
#14019=CARTESIAN_POINT('Origin',(77.375,-3.3,34.25)) ;
#14020=CARTESIAN_POINT('Origin',(-38.,-43.8,31.)) ;
#14021=CARTESIAN_POINT('',(-81.25,-49.3,31.)) ;
#14022=CARTESIAN_POINT('',(-81.25,-38.3,31.)) ;
#14023=CARTESIAN_POINT('',(-81.25,-46.55,31.)) ;
#14024=CARTESIAN_POINT('',(6.,-49.3,31.)) ;
#14025=CARTESIAN_POINT('',(24.625,-49.3,31.)) ;
#14026=CARTESIAN_POINT('',(6.,-38.3,31.)) ;
#14027=CARTESIAN_POINT('',(6.,-49.3,31.)) ;
#14028=CARTESIAN_POINT('',(6.,-38.3,31.)) ;
#14029=CARTESIAN_POINT('Origin',(6.,-38.3,29.1)) ;
#14030=CARTESIAN_POINT('',(-81.25,-38.3,29.1)) ;
#14031=CARTESIAN_POINT('',(-81.25,-38.3,29.1)) ;
#14032=CARTESIAN_POINT('',(6.,-38.3,29.1)) ;
#14033=CARTESIAN_POINT('',(6.,-38.3,29.1)) ;
#14034=CARTESIAN_POINT('',(6.,-38.3,29.1)) ;
#14035=CARTESIAN_POINT('Origin',(6.,-49.3,29.1)) ;
#14036=CARTESIAN_POINT('',(6.,-49.3,29.1)) ;
#14037=CARTESIAN_POINT('',(6.,-49.3,29.1)) ;
#14038=CARTESIAN_POINT('',(6.,-49.3,29.1)) ;
#14039=CARTESIAN_POINT('Origin',(84.25,45.,46.8)) ;
#14040=CARTESIAN_POINT('',(80.25,45.,55.)) ;
#14041=CARTESIAN_POINT('Origin',(84.25,45.,55.)) ;
#14042=CARTESIAN_POINT('',(80.25,45.,38.6)) ;
#14043=CARTESIAN_POINT('',(80.25,45.,46.8)) ;
#14044=CARTESIAN_POINT('Origin',(84.25,45.,38.6)) ;
#14045=CARTESIAN_POINT('Origin',(84.25,45.,38.6)) ;
#14046=CARTESIAN_POINT('Origin',(84.25,45.,39.1)) ;
#14047=CARTESIAN_POINT('Origin',(84.25,45.,38.6)) ;
#14048=CARTESIAN_POINT('Origin',(88.25,45.,38.6)) ;
#14049=CARTESIAN_POINT('Origin',(88.25,45.,38.6)) ;
#14050=CARTESIAN_POINT('Origin',(84.25,45.,55.)) ;
#14051=CARTESIAN_POINT('Origin',(81.25,2.3,30.)) ;
#14052=CARTESIAN_POINT('',(81.25,2.3,30.)) ;
#14053=CARTESIAN_POINT('Origin',(80.5,2.3,35.)) ;
#14054=CARTESIAN_POINT('',(80.5,2.3,35.)) ;
#14055=CARTESIAN_POINT('',(80.5,2.3,35.)) ;
#14056=CARTESIAN_POINT('',(80.5,2.3,35.)) ;
#14057=CARTESIAN_POINT('Origin',(77.,2.3,35.)) ;
#14058=CARTESIAN_POINT('Origin',(77.,2.3,35.)) ;
#14059=CARTESIAN_POINT('Origin',(77.375,2.3,34.25)) ;
#14060=CARTESIAN_POINT('Origin',(-38.,43.8,31.)) ;
#14061=CARTESIAN_POINT('',(-81.25,38.3,31.)) ;
#14062=CARTESIAN_POINT('',(-81.25,49.3,31.)) ;
#14063=CARTESIAN_POINT('',(-81.25,-2.75,31.)) ;
#14064=CARTESIAN_POINT('',(6.,38.3,31.)) ;
#14065=CARTESIAN_POINT('',(-82.,38.3,31.)) ;
#14066=CARTESIAN_POINT('',(6.,49.3,31.)) ;
#14067=CARTESIAN_POINT('',(6.,38.3,31.)) ;
#14068=CARTESIAN_POINT('',(-62.625,49.3,31.)) ;
#14069=CARTESIAN_POINT('Origin',(-82.,38.3,29.1)) ;
#14070=CARTESIAN_POINT('',(-81.25,38.3,29.1)) ;
#14071=CARTESIAN_POINT('',(-81.25,38.3,29.1)) ;
#14072=CARTESIAN_POINT('',(6.,38.3,29.1)) ;
#14073=CARTESIAN_POINT('',(-82.,38.3,29.1)) ;
#14074=CARTESIAN_POINT('',(6.,38.3,29.1)) ;
#14075=CARTESIAN_POINT('Origin',(6.,38.3,29.1)) ;
#14076=CARTESIAN_POINT('',(6.,49.3,29.1)) ;
#14077=CARTESIAN_POINT('',(6.,38.3,29.1)) ;
#14078=CARTESIAN_POINT('',(6.,49.3,29.1)) ;
#14079=CARTESIAN_POINT('Origin',(-78.25,-52.3,29.1)) ;
#14080=CARTESIAN_POINT('',(-87.25,-59.3,29.1)) ;
#14081=CARTESIAN_POINT('',(-87.25,-45.3,29.1)) ;
#14082=CARTESIAN_POINT('',(-69.25,-59.3,29.1)) ;
#14083=CARTESIAN_POINT('',(-87.25,-59.3,29.1)) ;
#14084=CARTESIAN_POINT('',(-69.25,-59.3,29.1)) ;
#14085=CARTESIAN_POINT('Origin',(-69.25,-45.3,27.6)) ;
#14086=CARTESIAN_POINT('',(-87.25,-45.3,29.1)) ;
#14087=CARTESIAN_POINT('',(-87.25,-45.3,27.6)) ;
#14088=CARTESIAN_POINT('',(-69.25,-45.3,29.1)) ;
#14089=CARTESIAN_POINT('',(-34.625,-45.3,29.1)) ;
#14090=CARTESIAN_POINT('',(-69.25,-45.3,27.6)) ;
#14091=CARTESIAN_POINT('Origin',(-69.25,-59.3,27.6)) ;
#14092=CARTESIAN_POINT('',(-69.25,-59.3,29.1)) ;
#14093=CARTESIAN_POINT('',(-69.25,-59.3,27.6)) ;
#14094=CARTESIAN_POINT('Origin',(-87.25,-59.3,27.6)) ;
#14095=CARTESIAN_POINT('',(-87.25,-59.3,27.6)) ;
#14096=CARTESIAN_POINT('Origin',(-78.25,52.3,29.1)) ;
#14097=CARTESIAN_POINT('',(-69.25,59.3,29.1)) ;
#14098=CARTESIAN_POINT('',(-69.25,45.3,29.1)) ;
#14099=CARTESIAN_POINT('',(-87.25,59.3,29.1)) ;
#14100=CARTESIAN_POINT('',(-69.25,59.3,29.1)) ;
#14101=CARTESIAN_POINT('',(-87.25,59.3,29.1)) ;
#14102=CARTESIAN_POINT('Origin',(-69.25,59.3,27.6)) ;
#14103=CARTESIAN_POINT('',(-87.25,59.3,27.6)) ;
#14104=CARTESIAN_POINT('',(-69.25,59.3,27.6)) ;
#14105=CARTESIAN_POINT('Origin',(-69.25,45.3,27.6)) ;
#14106=CARTESIAN_POINT('',(-69.25,45.3,29.1)) ;
#14107=CARTESIAN_POINT('',(-69.25,48.8,29.1)) ;
#14108=CARTESIAN_POINT('',(-69.25,45.3,27.6)) ;
#14109=CARTESIAN_POINT('Origin',(-87.25,45.3,27.6)) ;
#14110=CARTESIAN_POINT('',(-87.25,45.3,29.1)) ;
#14111=CARTESIAN_POINT('',(-87.25,45.3,29.1)) ;
#14112=CARTESIAN_POINT('',(-87.25,45.3,27.6)) ;
#14113=CARTESIAN_POINT('Origin',(0.,52.3,29.1)) ;
#14114=CARTESIAN_POINT('',(-87.25,55.3,29.1)) ;
#14115=CARTESIAN_POINT('',(69.25,49.3,29.1)) ;
#14116=CARTESIAN_POINT('',(69.25,55.8,29.1)) ;
#14117=CARTESIAN_POINT('',(-87.25,49.3,29.1)) ;
#14118=CARTESIAN_POINT('',(-81.25,-49.3,29.1)) ;
#14119=CARTESIAN_POINT('',(69.25,-49.3,29.1)) ;
#14120=CARTESIAN_POINT('',(87.25,-49.3,29.1)) ;
#14121=CARTESIAN_POINT('',(69.25,3.5,29.1)) ;
#14122=CARTESIAN_POINT('Origin',(-81.25,-49.3,29.1)) ;
#14123=CARTESIAN_POINT('',(-81.25,49.3,39.1)) ;
#14124=CARTESIAN_POINT('',(-81.25,49.3,29.1)) ;
#14125=CARTESIAN_POINT('',(-81.25,-49.3,39.1)) ;
#14126=CARTESIAN_POINT('',(-81.25,-49.3,39.1)) ;
#14127=CARTESIAN_POINT('',(-81.25,-49.3,29.1)) ;
#14128=CARTESIAN_POINT('Origin',(-87.25,49.3,29.1)) ;
#14129=CARTESIAN_POINT('',(-87.25,49.3,29.1)) ;
#14130=CARTESIAN_POINT('',(-87.25,49.3,39.1)) ;
#14131=CARTESIAN_POINT('Origin',(78.25,-52.3,29.1)) ;
#14132=CARTESIAN_POINT('',(69.25,-59.3,29.1)) ;
#14133=CARTESIAN_POINT('',(69.25,-45.3,29.1)) ;
#14134=CARTESIAN_POINT('',(69.25,-59.3,29.1)) ;
#14135=CARTESIAN_POINT('Origin',(87.25,-45.3,27.6)) ;
#14136=CARTESIAN_POINT('',(69.25,-45.3,29.1)) ;
#14137=CARTESIAN_POINT('',(69.25,-45.3,27.6)) ;
#14138=CARTESIAN_POINT('',(87.25,-45.3,29.1)) ;
#14139=CARTESIAN_POINT('',(43.625,-45.3,29.1)) ;
#14140=CARTESIAN_POINT('Origin',(69.25,-59.3,27.6)) ;
#14141=CARTESIAN_POINT('',(69.25,-59.3,27.6)) ;
#14142=CARTESIAN_POINT('Origin',(69.25,-45.3,27.6)) ;
#14143=CARTESIAN_POINT('',(69.25,-45.3,29.1)) ;
#14144=CARTESIAN_POINT('Origin',(78.25,-52.3,29.1)) ;
#14145=CARTESIAN_POINT('',(87.25,-49.3,29.1)) ;
#14146=CARTESIAN_POINT('Origin',(0.,52.3,29.1)) ;
#14147=CARTESIAN_POINT('',(34.625,45.3,29.1)) ;
#14148=CARTESIAN_POINT('Origin',(78.25,52.3,29.1)) ;
#14149=CARTESIAN_POINT('',(69.25,59.3,29.1)) ;
#14150=CARTESIAN_POINT('',(87.25,59.3,29.1)) ;
#14151=CARTESIAN_POINT('',(69.25,59.3,29.1)) ;
#14152=CARTESIAN_POINT('Origin',(78.25,52.3,29.1)) ;
#14153=CARTESIAN_POINT('',(69.25,45.3,29.1)) ;
#14154=CARTESIAN_POINT('',(69.25,59.3,29.1)) ;
#14155=CARTESIAN_POINT('',(69.25,45.3,29.1)) ;
#14156=CARTESIAN_POINT('Origin',(87.25,59.3,27.6)) ;
#14157=CARTESIAN_POINT('',(69.25,59.3,27.6)) ;
#14158=CARTESIAN_POINT('Origin',(69.25,45.3,27.6)) ;
#14159=CARTESIAN_POINT('',(69.25,45.3,27.6)) ;
#14160=CARTESIAN_POINT('Origin',(69.25,59.3,27.6)) ;
#14161=CARTESIAN_POINT('Origin',(87.25,-49.3,29.1)) ;
#14162=CARTESIAN_POINT('',(87.25,-49.3,39.1)) ;
#14163=CARTESIAN_POINT('Origin',(-87.25,55.3,29.1)) ;
#14164=CARTESIAN_POINT('',(-87.25,55.3,39.1)) ;
#14165=CARTESIAN_POINT('Origin',(0.,52.3,39.1)) ;
#18721=UNCERTAINTY_MEASURE_WITH_UNIT(LENGTH_MEASURE(0.01),#18758,
'DISTANCE_ACCURACY_VALUE',
'Maximum model space distance between geometric entities at asserted c
onnectivities') ;
#18738=UNCERTAINTY_MEASURE_WITH_UNIT(LENGTH_MEASURE(0.01),#18758,
'DISTANCE_ACCURACY_VALUE',
'Maximum model space distance between geometric entities at asserted c
onnectivities') ;
#18740=(
GEOMETRIC_REPRESENTATION_CONTEXT(3)
GLOBAL_UNCERTAINTY_ASSIGNED_CONTEXT((#18721))
GLOBAL_UNIT_ASSIGNED_CONTEXT((#18758,#18760,#18761))
REPRESENTATION_CONTEXT('','3D')
) ;
#18757=(
GEOMETRIC_REPRESENTATION_CONTEXT(3)
GLOBAL_UNCERTAINTY_ASSIGNED_CONTEXT((#18738))
GLOBAL_UNIT_ASSIGNED_CONTEXT((#18758,#18760,#18761))
REPRESENTATION_CONTEXT('','3D')
) ;
#18758=(
LENGTH_UNIT()
NAMED_UNIT(*)
SI_UNIT(.MILLI.,.METRE.)
) ;
#18760=(
NAMED_UNIT(*)
PLANE_ANGLE_UNIT()
SI_UNIT($,.RADIAN.)
) ;
#18761=(
NAMED_UNIT(*)
SI_UNIT($,.STERADIAN.)
SOLID_ANGLE_UNIT()
) ;
#18763=SHAPE_DEFINITION_REPRESENTATION(#18781,#18857) ;
#18781=PRODUCT_DEFINITION_SHAPE('',$,#18876) ;
#18857=SHAPE_REPRESENTATION('',(#9748),#18740) ;
#18874=PRODUCT_DEFINITION_CONTEXT('part definition',#18930,'design') ;
#18876=PRODUCT_DEFINITION('Lift Table Base Frame Weldment',
'Lift Table Base Frame Weldment',#18894,#18874) ;
#18894=PRODUCT_DEFINITION_FORMATION('',$,#18933) ;
#18930=APPLICATION_CONTEXT(
'Core Data for Automotive Mechanical Design Process') ;
#18931=PRODUCT_CONTEXT('part definition',#18930,'mechanical') ;
#18933=PRODUCT('Lift Table Base Frame Weldment',
'Lift Table Base Frame Weldment',$,(#18931)) ;
#18951=PRESENTATION_STYLE_ASSIGNMENT((#18969)) ;
#18969=SURFACE_STYLE_USAGE(.BOTH.,#18987) ;
#18987=SURFACE_SIDE_STYLE('',(#19005)) ;
#19005=SURFACE_STYLE_FILL_AREA(#19023) ;
#19023=FILL_AREA_STYLE(
'MAS-253 Metallic Sheet - Lift Table Base Frame Weldment',(#19041)) ;
#19041=FILL_AREA_STYLE_COLOUR(
'MAS-253 Metallic Sheet - Lift Table Base Frame Weldment',#19059) ;
#19059=COLOUR_RGB(
'MAS-253 Metallic Sheet - Lift Table Base Frame Weldment', 0.66274510, 0.83137255, 0.94901961) ;
ENDSEC;
END-ISO-10303-21;
